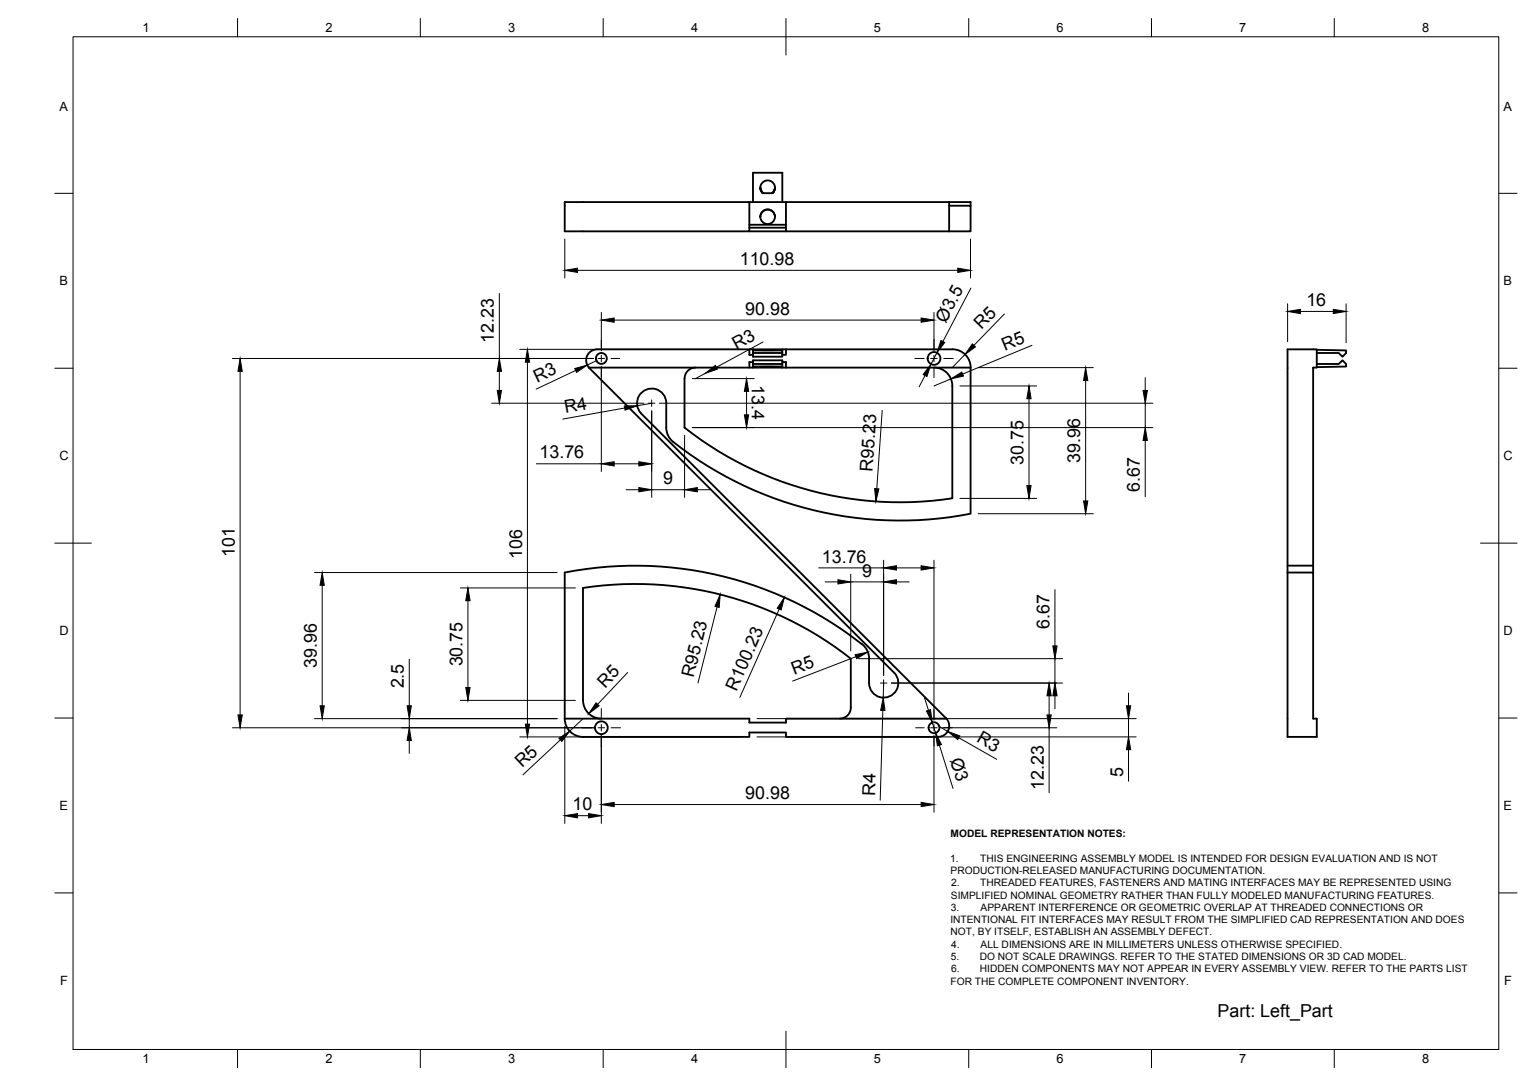
ISO-10303-21;
HEADER;
/* Generated by software containing ST-Developer
 * from STEP Tools, Inc. (www.steptools.com) 
 */

FILE_DESCRIPTION(
/* description */ (''),
/* implementation_level */ '2;1');

FILE_NAME(
/* name */ 'Left_Part.step',
/* time_stamp */ '2026-10-05T13:12:53-07:00',
/* author */ (''),
/* organization */ (''),
/* preprocessor_version */ 'ST-DEVELOPER v20.2',
/* originating_system */ 'Autodesk Translation Framework v15.15.0.0',
/* authorisation */ '');

FILE_SCHEMA (('AUTOMOTIVE_DESIGN { 1 0 10303 214 3 1 1 }'));
ENDSEC;

DATA;
#10=MECHANICAL_DESIGN_GEOMETRIC_PRESENTATION_REPRESENTATION('',(#59),#5912);
#43=SHAPE_REPRESENTATION_RELATIONSHIP('SRR','None',#5944,#51);
#51=ADVANCED_BREP_SHAPE_REPRESENTATION('',(#67),#5904);
#59=STYLED_ITEM('',(#5993),#67);
#67=MANIFOLD_SOLID_BREP('Body1',#3470);
#75=FACE_BOUND('',#374,.T.);
#76=FACE_BOUND('',#375,.T.);
#77=FACE_BOUND('',#379,.T.);
#78=FACE_BOUND('',#419,.T.);
#79=FACE_BOUND('',#421,.T.);
#80=FACE_BOUND('',#427,.T.);
#81=FACE_BOUND('',#428,.T.);
#82=FACE_BOUND('',#432,.T.);
#83=FACE_BOUND('',#437,.T.);
#84=FACE_BOUND('',#441,.T.);
#85=FACE_BOUND('',#442,.T.);
#96=ELLIPSE('',#3572,2.00043399581457,2.);
#97=ELLIPSE('',#3573,2.00173692551084,2.);
#98=ELLIPSE('',#3574,2.00173692551084,2.);
#99=ELLIPSE('',#3577,2.00043399581457,2.);
#100=ELLIPSE('',#3579,2.00043399581457,2.);
#101=ELLIPSE('',#3580,2.77129645175522,2.);
#102=ELLIPSE('',#3581,2.00043399581457,2.);
#103=ELLIPSE('',#3582,2.00043399581457,2.);
#114=CYLINDRICAL_SURFACE('',#3571,2.);
#115=CYLINDRICAL_SURFACE('',#3575,2.);
#116=CYLINDRICAL_SURFACE('',#3578,2.);
#117=CYLINDRICAL_SURFACE('',#3584,1.50000013517123);
#118=CYLINDRICAL_SURFACE('',#3588,1.4999996247669);
#119=CYLINDRICAL_SURFACE('',#3597,1.74999969554324);
#120=CYLINDRICAL_SURFACE('',#3601,4.99999999999999);
#121=CYLINDRICAL_SURFACE('',#3604,5.);
#122=CYLINDRICAL_SURFACE('',#3614,100.231846914414);
#123=CYLINDRICAL_SURFACE('',#3621,3.00000000000007);
#124=CYLINDRICAL_SURFACE('',#3625,95.2318469144141);
#125=CYLINDRICAL_SURFACE('',#3629,5.00000220964233);
#126=CYLINDRICAL_SURFACE('',#3633,3.99998589024062);
#127=CYLINDRICAL_SURFACE('',#3637,2.99999999999999);
#128=CYLINDRICAL_SURFACE('',#3640,3.00000000000001);
#129=CYLINDRICAL_SURFACE('',#3645,3.99998589024062);
#130=CYLINDRICAL_SURFACE('',#3649,5.00000220964233);
#131=CYLINDRICAL_SURFACE('',#3653,3.00000000000008);
#132=CYLINDRICAL_SURFACE('',#3656,2.99999999999999);
#133=CYLINDRICAL_SURFACE('',#3663,100.231846914414);
#134=CYLINDRICAL_SURFACE('',#3667,5.);
#135=CYLINDRICAL_SURFACE('',#3671,5.);
#136=CYLINDRICAL_SURFACE('',#3677,1.75000228959638);
#137=CYLINDRICAL_SURFACE('',#3694,95.231846914414);
#168=FACE_OUTER_BOUND('',#350,.T.);
#169=FACE_OUTER_BOUND('',#351,.T.);
#170=FACE_OUTER_BOUND('',#352,.T.);
#171=FACE_OUTER_BOUND('',#353,.T.);
#172=FACE_OUTER_BOUND('',#354,.T.);
#173=FACE_OUTER_BOUND('',#355,.T.);
#174=FACE_OUTER_BOUND('',#356,.T.);
#175=FACE_OUTER_BOUND('',#357,.T.);
#176=FACE_OUTER_BOUND('',#358,.T.);
#177=FACE_OUTER_BOUND('',#359,.T.);
#178=FACE_OUTER_BOUND('',#360,.T.);
#179=FACE_OUTER_BOUND('',#361,.T.);
#180=FACE_OUTER_BOUND('',#362,.T.);
#181=FACE_OUTER_BOUND('',#363,.T.);
#182=FACE_OUTER_BOUND('',#364,.T.);
#183=FACE_OUTER_BOUND('',#365,.T.);
#184=FACE_OUTER_BOUND('',#366,.T.);
#185=FACE_OUTER_BOUND('',#367,.T.);
#186=FACE_OUTER_BOUND('',#368,.T.);
#187=FACE_OUTER_BOUND('',#369,.T.);
#188=FACE_OUTER_BOUND('',#370,.T.);
#189=FACE_OUTER_BOUND('',#371,.T.);
#190=FACE_OUTER_BOUND('',#372,.T.);
#191=FACE_OUTER_BOUND('',#373,.T.);
#192=FACE_OUTER_BOUND('',#376,.T.);
#193=FACE_OUTER_BOUND('',#377,.T.);
#194=FACE_OUTER_BOUND('',#378,.T.);
#195=FACE_OUTER_BOUND('',#380,.T.);
#196=FACE_OUTER_BOUND('',#381,.T.);
#197=FACE_OUTER_BOUND('',#382,.T.);
#198=FACE_OUTER_BOUND('',#383,.T.);
#199=FACE_OUTER_BOUND('',#384,.T.);
#200=FACE_OUTER_BOUND('',#385,.T.);
#201=FACE_OUTER_BOUND('',#386,.T.);
#202=FACE_OUTER_BOUND('',#387,.T.);
#203=FACE_OUTER_BOUND('',#388,.T.);
#204=FACE_OUTER_BOUND('',#389,.T.);
#205=FACE_OUTER_BOUND('',#390,.T.);
#206=FACE_OUTER_BOUND('',#391,.T.);
#207=FACE_OUTER_BOUND('',#392,.T.);
#208=FACE_OUTER_BOUND('',#393,.T.);
#209=FACE_OUTER_BOUND('',#394,.T.);
#210=FACE_OUTER_BOUND('',#395,.T.);
#211=FACE_OUTER_BOUND('',#396,.T.);
#212=FACE_OUTER_BOUND('',#397,.T.);
#213=FACE_OUTER_BOUND('',#398,.T.);
#214=FACE_OUTER_BOUND('',#399,.T.);
#215=FACE_OUTER_BOUND('',#400,.T.);
#216=FACE_OUTER_BOUND('',#401,.T.);
#217=FACE_OUTER_BOUND('',#402,.T.);
#218=FACE_OUTER_BOUND('',#403,.T.);
#219=FACE_OUTER_BOUND('',#404,.T.);
#220=FACE_OUTER_BOUND('',#405,.T.);
#221=FACE_OUTER_BOUND('',#406,.T.);
#222=FACE_OUTER_BOUND('',#407,.T.);
#223=FACE_OUTER_BOUND('',#408,.T.);
#224=FACE_OUTER_BOUND('',#409,.T.);
#225=FACE_OUTER_BOUND('',#410,.T.);
#226=FACE_OUTER_BOUND('',#411,.T.);
#227=FACE_OUTER_BOUND('',#412,.T.);
#228=FACE_OUTER_BOUND('',#413,.T.);
#229=FACE_OUTER_BOUND('',#414,.T.);
#230=FACE_OUTER_BOUND('',#415,.T.);
#231=FACE_OUTER_BOUND('',#416,.T.);
#232=FACE_OUTER_BOUND('',#417,.T.);
#233=FACE_OUTER_BOUND('',#418,.T.);
#234=FACE_OUTER_BOUND('',#420,.T.);
#235=FACE_OUTER_BOUND('',#422,.T.);
#236=FACE_OUTER_BOUND('',#423,.T.);
#237=FACE_OUTER_BOUND('',#424,.T.);
#238=FACE_OUTER_BOUND('',#425,.T.);
#239=FACE_OUTER_BOUND('',#426,.T.);
#240=FACE_OUTER_BOUND('',#429,.T.);
#241=FACE_OUTER_BOUND('',#430,.T.);
#242=FACE_OUTER_BOUND('',#431,.T.);
#243=FACE_OUTER_BOUND('',#433,.T.);
#244=FACE_OUTER_BOUND('',#434,.T.);
#245=FACE_OUTER_BOUND('',#435,.T.);
#246=FACE_OUTER_BOUND('',#436,.T.);
#247=FACE_OUTER_BOUND('',#438,.T.);
#248=FACE_OUTER_BOUND('',#439,.T.);
#249=FACE_OUTER_BOUND('',#440,.T.);
#350=EDGE_LOOP('',(#2190,#2191));
#351=EDGE_LOOP('',(#2192,#2193,#2194,#2195,#2196,#2197));
#352=EDGE_LOOP('',(#2198,#2199,#2200,#2201));
#353=EDGE_LOOP('',(#2202,#2203,#2204,#2205,#2206,#2207));
#354=EDGE_LOOP('',(#2208,#2209,#2210,#2211,#2212,#2213,#2214));
#355=EDGE_LOOP('',(#2215,#2216,#2217,#2218));
#356=EDGE_LOOP('',(#2219));
#357=EDGE_LOOP('',(#2220,#2221,#2222,#2223));
#358=EDGE_LOOP('',(#2224));
#359=EDGE_LOOP('',(#2225,#2226,#2227,#2228,#2229,#2230));
#360=EDGE_LOOP('',(#2231,#2232,#2233,#2234,#2235,#2236));
#361=EDGE_LOOP('',(#2237,#2238,#2239,#2240,#2241));
#362=EDGE_LOOP('',(#2242));
#363=EDGE_LOOP('',(#2243,#2244,#2245,#2246));
#364=EDGE_LOOP('',(#2247,#2248,#2249,#2250,#2251,#2252));
#365=EDGE_LOOP('',(#2253,#2254,#2255,#2256));
#366=EDGE_LOOP('',(#2257,#2258,#2259,#2260));
#367=EDGE_LOOP('',(#2261,#2262,#2263,#2264,#2265,#2266));
#368=EDGE_LOOP('',(#2267,#2268,#2269,#2270));
#369=EDGE_LOOP('',(#2271,#2272,#2273,#2274));
#370=EDGE_LOOP('',(#2275,#2276,#2277,#2278));
#371=EDGE_LOOP('',(#2279,#2280,#2281,#2282,#2283,#2284));
#372=EDGE_LOOP('',(#2285,#2286,#2287,#2288));
#373=EDGE_LOOP('',(#2289,#2290,#2291,#2292,#2293,#2294,#2295,#2296,#2297,
#2298,#2299,#2300));
#374=EDGE_LOOP('',(#2301));
#375=EDGE_LOOP('',(#2302));
#376=EDGE_LOOP('',(#2303,#2304,#2305,#2306));
#377=EDGE_LOOP('',(#2307,#2308,#2309,#2310,#2311,#2312));
#378=EDGE_LOOP('',(#2313,#2314,#2315,#2316));
#379=EDGE_LOOP('',(#2317));
#380=EDGE_LOOP('',(#2318,#2319,#2320,#2321,#2322,#2323));
#381=EDGE_LOOP('',(#2324,#2325,#2326,#2327,#2328,#2329));
#382=EDGE_LOOP('',(#2330,#2331,#2332,#2333));
#383=EDGE_LOOP('',(#2334,#2335,#2336,#2337));
#384=EDGE_LOOP('',(#2338,#2339,#2340,#2341));
#385=EDGE_LOOP('',(#2342,#2343,#2344,#2345));
#386=EDGE_LOOP('',(#2346,#2347,#2348,#2349));
#387=EDGE_LOOP('',(#2350,#2351,#2352,#2353));
#388=EDGE_LOOP('',(#2354,#2355,#2356,#2357));
#389=EDGE_LOOP('',(#2358,#2359,#2360,#2361,#2362));
#390=EDGE_LOOP('',(#2363,#2364,#2365,#2366,#2367,#2368,#2369));
#391=EDGE_LOOP('',(#2370,#2371,#2372,#2373,#2374));
#392=EDGE_LOOP('',(#2375,#2376,#2377,#2378));
#393=EDGE_LOOP('',(#2379,#2380,#2381,#2382));
#394=EDGE_LOOP('',(#2383,#2384,#2385,#2386));
#395=EDGE_LOOP('',(#2387,#2388,#2389,#2390));
#396=EDGE_LOOP('',(#2391,#2392,#2393,#2394));
#397=EDGE_LOOP('',(#2395,#2396,#2397,#2398));
#398=EDGE_LOOP('',(#2399,#2400,#2401,#2402));
#399=EDGE_LOOP('',(#2403,#2404,#2405,#2406));
#400=EDGE_LOOP('',(#2407,#2408,#2409,#2410));
#401=EDGE_LOOP('',(#2411,#2412,#2413,#2414,#2415,#2416));
#402=EDGE_LOOP('',(#2417,#2418,#2419,#2420,#2421,#2422));
#403=EDGE_LOOP('',(#2423,#2424,#2425,#2426));
#404=EDGE_LOOP('',(#2427,#2428,#2429,#2430));
#405=EDGE_LOOP('',(#2431,#2432,#2433,#2434));
#406=EDGE_LOOP('',(#2435,#2436,#2437,#2438,#2439));
#407=EDGE_LOOP('',(#2440,#2441,#2442,#2443,#2444,#2445,#2446,#2447,#2448,
#2449,#2450));
#408=EDGE_LOOP('',(#2451,#2452,#2453,#2454));
#409=EDGE_LOOP('',(#2455,#2456,#2457,#2458));
#410=EDGE_LOOP('',(#2459,#2460,#2461,#2462,#2463,#2464,#2465,#2466,#2467,
#2468,#2469,#2470,#2471,#2472,#2473,#2474,#2475,#2476,#2477,#2478,#2479,
#2480,#2481,#2482,#2483,#2484,#2485,#2486,#2487));
#411=EDGE_LOOP('',(#2488,#2489,#2490,#2491));
#412=EDGE_LOOP('',(#2492));
#413=EDGE_LOOP('',(#2493,#2494,#2495,#2496));
#414=EDGE_LOOP('',(#2497,#2498,#2499,#2500,#2501,#2502,#2503,#2504));
#415=EDGE_LOOP('',(#2505,#2506,#2507,#2508));
#416=EDGE_LOOP('',(#2509,#2510,#2511,#2512));
#417=EDGE_LOOP('',(#2513,#2514,#2515,#2516));
#418=EDGE_LOOP('',(#2517,#2518,#2519,#2520));
#419=EDGE_LOOP('',(#2521));
#420=EDGE_LOOP('',(#2522,#2523,#2524,#2525));
#421=EDGE_LOOP('',(#2526));
#422=EDGE_LOOP('',(#2527,#2528,#2529,#2530));
#423=EDGE_LOOP('',(#2531,#2532,#2533,#2534));
#424=EDGE_LOOP('',(#2535,#2536,#2537,#2538,#2539,#2540));
#425=EDGE_LOOP('',(#2541,#2542,#2543,#2544,#2545,#2546));
#426=EDGE_LOOP('',(#2547,#2548,#2549,#2550,#2551,#2552,#2553,#2554,#2555,
#2556,#2557,#2558,#2559,#2560,#2561,#2562,#2563,#2564,#2565,#2566,#2567,
#2568,#2569));
#427=EDGE_LOOP('',(#2570,#2571,#2572,#2573,#2574,#2575,#2576,#2577,#2578,
#2579));
#428=EDGE_LOOP('',(#2580,#2581,#2582,#2583,#2584,#2585));
#429=EDGE_LOOP('',(#2586,#2587,#2588,#2589));
#430=EDGE_LOOP('',(#2590,#2591,#2592,#2593,#2594,#2595,#2596,#2597,#2598,
#2599,#2600,#2601,#2602,#2603));
#431=EDGE_LOOP('',(#2604,#2605,#2606,#2607));
#432=EDGE_LOOP('',(#2608,#2609,#2610));
#433=EDGE_LOOP('',(#2611,#2612,#2613,#2614));
#434=EDGE_LOOP('',(#2615,#2616,#2617,#2618));
#435=EDGE_LOOP('',(#2619,#2620,#2621,#2622));
#436=EDGE_LOOP('',(#2623,#2624,#2625,#2626));
#437=EDGE_LOOP('',(#2627));
#438=EDGE_LOOP('',(#2628,#2629,#2630,#2631,#2632,#2633,#2634,#2635));
#439=EDGE_LOOP('',(#2636,#2637,#2638,#2639));
#440=EDGE_LOOP('',(#2640,#2641,#2642,#2643,#2644,#2645,#2646,#2647,#2648,
#2649,#2650,#2651));
#441=EDGE_LOOP('',(#2652));
#442=EDGE_LOOP('',(#2653));
#553=CIRCLE('',#3570,2.);
#554=CIRCLE('',#3576,2.);
#555=CIRCLE('',#3585,1.50000013517123);
#556=CIRCLE('',#3586,1.50000013517123);
#557=CIRCLE('',#3589,1.4999996247669);
#558=CIRCLE('',#3590,1.4999996247669);
#559=CIRCLE('',#3596,1.74999969554324);
#560=CIRCLE('',#3598,1.74999969554324);
#561=CIRCLE('',#3602,4.99999999999999);
#562=CIRCLE('',#3603,4.99999999999999);
#563=CIRCLE('',#3605,5.);
#564=CIRCLE('',#3606,5.);
#565=CIRCLE('',#3613,2.99999999999999);
#566=CIRCLE('',#3615,100.231846914414);
#567=CIRCLE('',#3616,100.231846914414);
#568=CIRCLE('',#3622,3.00000000000007);
#569=CIRCLE('',#3623,3.00000000000007);
#570=CIRCLE('',#3626,95.2318469144141);
#571=CIRCLE('',#3627,95.2318469144141);
#572=CIRCLE('',#3630,5.00000220964233);
#573=CIRCLE('',#3631,5.00000220964233);
#574=CIRCLE('',#3634,3.99998589024062);
#575=CIRCLE('',#3635,3.99998589024062);
#576=CIRCLE('',#3638,2.99999999999999);
#577=CIRCLE('',#3639,2.99999999999999);
#578=CIRCLE('',#3641,3.00000000000001);
#579=CIRCLE('',#3642,3.00000000000001);
#580=CIRCLE('',#3643,3.00000000000001);
#581=CIRCLE('',#3646,3.99998589024062);
#582=CIRCLE('',#3647,3.99998589024062);
#583=CIRCLE('',#3650,5.00000220964233);
#584=CIRCLE('',#3651,5.00000220964233);
#585=CIRCLE('',#3654,3.00000000000008);
#586=CIRCLE('',#3655,3.00000000000008);
#587=CIRCLE('',#3657,2.99999999999999);
#588=CIRCLE('',#3664,100.231846914414);
#589=CIRCLE('',#3665,100.231846914414);
#590=CIRCLE('',#3668,5.);
#591=CIRCLE('',#3669,5.);
#592=CIRCLE('',#3672,5.);
#593=CIRCLE('',#3673,5.);
#594=CIRCLE('',#3676,95.231846914414);
#595=CIRCLE('',#3678,1.75000228959638);
#596=CIRCLE('',#3679,1.75000228959638);
#597=CIRCLE('',#3693,95.231846914414);
#655=LINE('',#4894,#1020);
#656=LINE('',#4900,#1021);
#657=LINE('',#4907,#1022);
#658=LINE('',#4917,#1023);
#659=LINE('',#4921,#1024);
#660=LINE('',#4923,#1025);
#661=LINE('',#4925,#1026);
#662=LINE('',#4927,#1027);
#663=LINE('',#4928,#1028);
#664=LINE('',#4933,#1029);
#665=LINE('',#4940,#1030);
#666=LINE('',#4945,#1031);
#667=LINE('',#4947,#1032);
#668=LINE('',#4949,#1033);
#669=LINE('',#4951,#1034);
#670=LINE('',#4952,#1035);
#671=LINE('',#4956,#1036);
#672=LINE('',#4958,#1037);
#673=LINE('',#4960,#1038);
#674=LINE('',#4962,#1039);
#675=LINE('',#4964,#1040);
#676=LINE('',#4965,#1041);
#677=LINE('',#4968,#1042);
#678=LINE('',#4970,#1043);
#679=LINE('',#4972,#1044);
#680=LINE('',#4973,#1045);
#681=LINE('',#4979,#1046);
#682=LINE('',#4983,#1047);
#683=LINE('',#4985,#1048);
#684=LINE('',#4987,#1049);
#685=LINE('',#4989,#1050);
#686=LINE('',#4990,#1051);
#687=LINE('',#4994,#1052);
#688=LINE('',#4996,#1053);
#689=LINE('',#4998,#1054);
#690=LINE('',#4999,#1055);
#691=LINE('',#5007,#1056);
#692=LINE('',#5010,#1057);
#693=LINE('',#5012,#1058);
#694=LINE('',#5013,#1059);
#695=LINE('',#5016,#1060);
#696=LINE('',#5018,#1061);
#697=LINE('',#5019,#1062);
#698=LINE('',#5022,#1063);
#699=LINE('',#5023,#1064);
#700=LINE('',#5026,#1065);
#701=LINE('',#5027,#1066);
#702=LINE('',#5030,#1067);
#703=LINE('',#5031,#1068);
#704=LINE('',#5034,#1069);
#705=LINE('',#5036,#1070);
#706=LINE('',#5038,#1071);
#707=LINE('',#5042,#1072);
#708=LINE('',#5043,#1073);
#709=LINE('',#5048,#1074);
#710=LINE('',#5052,#1075);
#711=LINE('',#5053,#1076);
#712=LINE('',#5055,#1077);
#713=LINE('',#5058,#1078);
#714=LINE('',#5059,#1079);
#715=LINE('',#5062,#1080);
#716=LINE('',#5064,#1081);
#717=LINE('',#5066,#1082);
#718=LINE('',#5067,#1083);
#719=LINE('',#5073,#1084);
#720=LINE('',#5076,#1085);
#721=LINE('',#5078,#1086);
#722=LINE('',#5079,#1087);
#723=LINE('',#5085,#1088);
#724=LINE('',#5087,#1089);
#725=LINE('',#5088,#1090);
#726=LINE('',#5094,#1091);
#727=LINE('',#5097,#1092);
#728=LINE('',#5099,#1093);
#729=LINE('',#5100,#1094);
#730=LINE('',#5106,#1095);
#731=LINE('',#5109,#1096);
#732=LINE('',#5111,#1097);
#733=LINE('',#5112,#1098);
#734=LINE('',#5117,#1099);
#735=LINE('',#5124,#1100);
#736=LINE('',#5129,#1101);
#737=LINE('',#5132,#1102);
#738=LINE('',#5134,#1103);
#739=LINE('',#5135,#1104);
#740=LINE('',#5140,#1105);
#741=LINE('',#5144,#1106);
#742=LINE('',#5146,#1107);
#743=LINE('',#5147,#1108);
#744=LINE('',#5152,#1109);
#745=LINE('',#5157,#1110);
#746=LINE('',#5159,#1111);
#747=LINE('',#5161,#1112);
#748=LINE('',#5162,#1113);
#749=LINE('',#5167,#1114);
#750=LINE('',#5171,#1115);
#751=LINE('',#5174,#1116);
#752=LINE('',#5178,#1117);
#753=LINE('',#5180,#1118);
#754=LINE('',#5182,#1119);
#755=LINE('',#5183,#1120);
#756=LINE('',#5187,#1121);
#757=LINE('',#5189,#1122);
#758=LINE('',#5191,#1123);
#759=LINE('',#5192,#1124);
#760=LINE('',#5196,#1125);
#761=LINE('',#5198,#1126);
#762=LINE('',#5200,#1127);
#763=LINE('',#5202,#1128);
#764=LINE('',#5204,#1129);
#765=LINE('',#5205,#1130);
#766=LINE('',#5209,#1131);
#767=LINE('',#5211,#1132);
#768=LINE('',#5213,#1133);
#769=LINE('',#5215,#1134);
#770=LINE('',#5217,#1135);
#771=LINE('',#5218,#1136);
#772=LINE('',#5220,#1137);
#773=LINE('',#5221,#1138);
#774=LINE('',#5226,#1139);
#775=LINE('',#5230,#1140);
#776=LINE('',#5232,#1141);
#777=LINE('',#5233,#1142);
#778=LINE('',#5238,#1143);
#779=LINE('',#5241,#1144);
#780=LINE('',#5244,#1145);
#781=LINE('',#5246,#1146);
#782=LINE('',#5248,#1147);
#783=LINE('',#5249,#1148);
#784=LINE('',#5250,#1149);
#785=LINE('',#5251,#1150);
#786=LINE('',#5252,#1151);
#787=LINE('',#5258,#1152);
#788=LINE('',#5261,#1153);
#789=LINE('',#5264,#1154);
#790=LINE('',#5266,#1155);
#791=LINE('',#5267,#1156);
#792=LINE('',#5269,#1157);
#793=LINE('',#5271,#1158);
#794=LINE('',#5276,#1159);
#795=LINE('',#5282,#1160);
#796=LINE('',#5284,#1161);
#797=LINE('',#5286,#1162);
#798=LINE('',#5287,#1163);
#799=LINE('',#5290,#1164);
#800=LINE('',#5291,#1165);
#801=LINE('',#5293,#1166);
#802=LINE('',#5294,#1167);
#803=LINE('',#5297,#1168);
#804=LINE('',#5298,#1169);
#805=LINE('',#5300,#1170);
#806=LINE('',#5303,#1171);
#807=LINE('',#5305,#1172);
#808=LINE('',#5306,#1173);
#809=LINE('',#5308,#1174);
#810=LINE('',#5311,#1175);
#811=LINE('',#5312,#1176);
#812=LINE('',#5315,#1177);
#813=LINE('',#5316,#1178);
#814=LINE('',#5318,#1179);
#815=LINE('',#5323,#1180);
#816=LINE('',#5325,#1181);
#817=LINE('',#5327,#1182);
#818=LINE('',#5329,#1183);
#819=LINE('',#5331,#1184);
#820=LINE('',#5332,#1185);
#821=LINE('',#5335,#1186);
#822=LINE('',#5338,#1187);
#823=LINE('',#5339,#1188);
#824=LINE('',#5340,#1189);
#825=LINE('',#5341,#1190);
#826=LINE('',#5342,#1191);
#827=LINE('',#5344,#1192);
#828=LINE('',#5346,#1193);
#829=LINE('',#5348,#1194);
#830=LINE('',#5350,#1195);
#831=LINE('',#5352,#1196);
#832=LINE('',#5354,#1197);
#833=LINE('',#5356,#1198);
#1020=VECTOR('',#3892,10.);
#1021=VECTOR('',#3899,2.);
#1022=VECTOR('',#3908,2.);
#1023=VECTOR('',#3919,2.);
#1024=VECTOR('',#3924,10.);
#1025=VECTOR('',#3925,10.);
#1026=VECTOR('',#3926,10.);
#1027=VECTOR('',#3927,10.);
#1028=VECTOR('',#3928,10.);
#1029=VECTOR('',#3933,1.50000013517123);
#1030=VECTOR('',#3942,1.4999996247669);
#1031=VECTOR('',#3949,10.);
#1032=VECTOR('',#3950,10.);
#1033=VECTOR('',#3951,10.);
#1034=VECTOR('',#3952,10.);
#1035=VECTOR('',#3953,10.);
#1036=VECTOR('',#3956,10.);
#1037=VECTOR('',#3957,10.);
#1038=VECTOR('',#3958,10.);
#1039=VECTOR('',#3959,10.);
#1040=VECTOR('',#3960,10.);
#1041=VECTOR('',#3961,10.);
#1042=VECTOR('',#3964,10.);
#1043=VECTOR('',#3965,10.);
#1044=VECTOR('',#3966,10.);
#1045=VECTOR('',#3967,10.);
#1046=VECTOR('',#3974,1.74999969554324);
#1047=VECTOR('',#3979,10.);
#1048=VECTOR('',#3980,10.);
#1049=VECTOR('',#3981,10.);
#1050=VECTOR('',#3982,10.);
#1051=VECTOR('',#3983,10.);
#1052=VECTOR('',#3986,10.);
#1053=VECTOR('',#3987,10.);
#1054=VECTOR('',#3988,10.);
#1055=VECTOR('',#3989,10.);
#1056=VECTOR('',#4002,10.);
#1057=VECTOR('',#4005,10.);
#1058=VECTOR('',#4006,10.);
#1059=VECTOR('',#4007,10.);
#1060=VECTOR('',#4010,10.);
#1061=VECTOR('',#4011,10.);
#1062=VECTOR('',#4012,10.);
#1063=VECTOR('',#4015,10.);
#1064=VECTOR('',#4016,10.);
#1065=VECTOR('',#4019,10.);
#1066=VECTOR('',#4020,10.);
#1067=VECTOR('',#4023,10.);
#1068=VECTOR('',#4024,10.);
#1069=VECTOR('',#4027,10.);
#1070=VECTOR('',#4028,10.);
#1071=VECTOR('',#4029,10.);
#1072=VECTOR('',#4032,10.);
#1073=VECTOR('',#4033,10.);
#1074=VECTOR('',#4038,10.);
#1075=VECTOR('',#4043,10.);
#1076=VECTOR('',#4044,10.);
#1077=VECTOR('',#4047,10.);
#1078=VECTOR('',#4050,10.);
#1079=VECTOR('',#4051,10.);
#1080=VECTOR('',#4054,10.);
#1081=VECTOR('',#4055,10.);
#1082=VECTOR('',#4056,10.);
#1083=VECTOR('',#4057,10.);
#1084=VECTOR('',#4064,10.);
#1085=VECTOR('',#4067,9.99999999999999);
#1086=VECTOR('',#4068,9.99999999999999);
#1087=VECTOR('',#4069,10.);
#1088=VECTOR('',#4078,10.);
#1089=VECTOR('',#4079,10.);
#1090=VECTOR('',#4080,10.);
#1091=VECTOR('',#4087,10.);
#1092=VECTOR('',#4090,10.);
#1093=VECTOR('',#4091,10.);
#1094=VECTOR('',#4092,10.);
#1095=VECTOR('',#4099,10.);
#1096=VECTOR('',#4102,10.);
#1097=VECTOR('',#4103,10.);
#1098=VECTOR('',#4104,10.);
#1099=VECTOR('',#4109,10.);
#1100=VECTOR('',#4116,10.);
#1101=VECTOR('',#4121,10.);
#1102=VECTOR('',#4124,10.);
#1103=VECTOR('',#4125,10.);
#1104=VECTOR('',#4126,10.);
#1105=VECTOR('',#4131,10.);
#1106=VECTOR('',#4136,10.);
#1107=VECTOR('',#4137,10.);
#1108=VECTOR('',#4138,10.);
#1109=VECTOR('',#4143,10.);
#1110=VECTOR('',#4148,9.99999999999999);
#1111=VECTOR('',#4149,10.);
#1112=VECTOR('',#4150,9.99999999999999);
#1113=VECTOR('',#4151,10.);
#1114=VECTOR('',#4156,10.);
#1115=VECTOR('',#4161,10.);
#1116=VECTOR('',#4164,10.);
#1117=VECTOR('',#4167,10.);
#1118=VECTOR('',#4168,10.);
#1119=VECTOR('',#4169,10.);
#1120=VECTOR('',#4170,10.);
#1121=VECTOR('',#4173,10.);
#1122=VECTOR('',#4174,10.);
#1123=VECTOR('',#4175,10.);
#1124=VECTOR('',#4176,10.);
#1125=VECTOR('',#4179,10.);
#1126=VECTOR('',#4180,10.);
#1127=VECTOR('',#4181,10.);
#1128=VECTOR('',#4182,10.);
#1129=VECTOR('',#4183,10.);
#1130=VECTOR('',#4184,10.);
#1131=VECTOR('',#4187,10.);
#1132=VECTOR('',#4188,10.);
#1133=VECTOR('',#4189,10.);
#1134=VECTOR('',#4190,10.);
#1135=VECTOR('',#4191,10.);
#1136=VECTOR('',#4192,10.);
#1137=VECTOR('',#4195,10.);
#1138=VECTOR('',#4196,10.);
#1139=VECTOR('',#4201,10.);
#1140=VECTOR('',#4206,10.);
#1141=VECTOR('',#4207,10.);
#1142=VECTOR('',#4208,10.);
#1143=VECTOR('',#4213,10.);
#1144=VECTOR('',#4216,10.);
#1145=VECTOR('',#4219,10.);
#1146=VECTOR('',#4220,10.);
#1147=VECTOR('',#4221,10.);
#1148=VECTOR('',#4222,10.);
#1149=VECTOR('',#4223,10.);
#1150=VECTOR('',#4224,10.);
#1151=VECTOR('',#4225,10.);
#1152=VECTOR('',#4230,10.);
#1153=VECTOR('',#4233,10.);
#1154=VECTOR('',#4236,10.);
#1155=VECTOR('',#4237,10.);
#1156=VECTOR('',#4238,10.);
#1157=VECTOR('',#4241,10.);
#1158=VECTOR('',#4244,10.);
#1159=VECTOR('',#4249,1.75000228959638);
#1160=VECTOR('',#4256,10.);
#1161=VECTOR('',#4257,10.);
#1162=VECTOR('',#4258,10.);
#1163=VECTOR('',#4259,10.);
#1164=VECTOR('',#4262,10.);
#1165=VECTOR('',#4263,10.);
#1166=VECTOR('',#4264,10.);
#1167=VECTOR('',#4265,10.);
#1168=VECTOR('',#4268,10.);
#1169=VECTOR('',#4269,10.);
#1170=VECTOR('',#4272,10.);
#1171=VECTOR('',#4275,10.);
#1172=VECTOR('',#4276,10.);
#1173=VECTOR('',#4277,10.);
#1174=VECTOR('',#4280,10.);
#1175=VECTOR('',#4283,10.);
#1176=VECTOR('',#4284,10.);
#1177=VECTOR('',#4287,10.);
#1178=VECTOR('',#4288,10.);
#1179=VECTOR('',#4291,10.);
#1180=VECTOR('',#4296,10.);
#1181=VECTOR('',#4297,10.);
#1182=VECTOR('',#4298,10.);
#1183=VECTOR('',#4299,10.);
#1184=VECTOR('',#4300,10.);
#1185=VECTOR('',#4301,10.);
#1186=VECTOR('',#4306,10.);
#1187=VECTOR('',#4311,10.);
#1188=VECTOR('',#4312,10.);
#1189=VECTOR('',#4313,10.);
#1190=VECTOR('',#4314,10.);
#1191=VECTOR('',#4315,10.);
#1192=VECTOR('',#4318,10.);
#1193=VECTOR('',#4321,10.);
#1194=VECTOR('',#4324,10.);
#1195=VECTOR('',#4327,10.);
#1196=VECTOR('',#4330,10.);
#1197=VECTOR('',#4333,10.);
#1198=VECTOR('',#4336,10.);
#1385=VERTEX_POINT('',#4892);
#1386=VERTEX_POINT('',#4893);
#1387=VERTEX_POINT('',#4897);
#1388=VERTEX_POINT('',#4899);
#1389=VERTEX_POINT('',#4904);
#1390=VERTEX_POINT('',#4906);
#1391=VERTEX_POINT('',#4910);
#1392=VERTEX_POINT('',#4911);
#1393=VERTEX_POINT('',#4913);
#1394=VERTEX_POINT('',#4916);
#1395=VERTEX_POINT('',#4920);
#1396=VERTEX_POINT('',#4922);
#1397=VERTEX_POINT('',#4924);
#1398=VERTEX_POINT('',#4926);
#1399=VERTEX_POINT('',#4930);
#1400=VERTEX_POINT('',#4932);
#1401=VERTEX_POINT('',#4937);
#1402=VERTEX_POINT('',#4939);
#1403=VERTEX_POINT('',#4944);
#1404=VERTEX_POINT('',#4946);
#1405=VERTEX_POINT('',#4948);
#1406=VERTEX_POINT('',#4950);
#1407=VERTEX_POINT('',#4954);
#1408=VERTEX_POINT('',#4955);
#1409=VERTEX_POINT('',#4957);
#1410=VERTEX_POINT('',#4959);
#1411=VERTEX_POINT('',#4961);
#1412=VERTEX_POINT('',#4963);
#1413=VERTEX_POINT('',#4967);
#1414=VERTEX_POINT('',#4969);
#1415=VERTEX_POINT('',#4971);
#1416=VERTEX_POINT('',#4975);
#1417=VERTEX_POINT('',#4978);
#1418=VERTEX_POINT('',#4982);
#1419=VERTEX_POINT('',#4984);
#1420=VERTEX_POINT('',#4986);
#1421=VERTEX_POINT('',#4988);
#1422=VERTEX_POINT('',#4992);
#1423=VERTEX_POINT('',#4993);
#1424=VERTEX_POINT('',#4995);
#1425=VERTEX_POINT('',#4997);
#1426=VERTEX_POINT('',#5004);
#1427=VERTEX_POINT('',#5009);
#1428=VERTEX_POINT('',#5011);
#1429=VERTEX_POINT('',#5015);
#1430=VERTEX_POINT('',#5017);
#1431=VERTEX_POINT('',#5021);
#1432=VERTEX_POINT('',#5025);
#1433=VERTEX_POINT('',#5029);
#1434=VERTEX_POINT('',#5033);
#1435=VERTEX_POINT('',#5035);
#1436=VERTEX_POINT('',#5037);
#1437=VERTEX_POINT('',#5039);
#1438=VERTEX_POINT('',#5041);
#1439=VERTEX_POINT('',#5045);
#1440=VERTEX_POINT('',#5047);
#1441=VERTEX_POINT('',#5051);
#1442=VERTEX_POINT('',#5057);
#1443=VERTEX_POINT('',#5061);
#1444=VERTEX_POINT('',#5063);
#1445=VERTEX_POINT('',#5065);
#1446=VERTEX_POINT('',#5069);
#1447=VERTEX_POINT('',#5071);
#1448=VERTEX_POINT('',#5075);
#1449=VERTEX_POINT('',#5077);
#1450=VERTEX_POINT('',#5084);
#1451=VERTEX_POINT('',#5086);
#1452=VERTEX_POINT('',#5090);
#1453=VERTEX_POINT('',#5092);
#1454=VERTEX_POINT('',#5096);
#1455=VERTEX_POINT('',#5098);
#1456=VERTEX_POINT('',#5102);
#1457=VERTEX_POINT('',#5104);
#1458=VERTEX_POINT('',#5108);
#1459=VERTEX_POINT('',#5110);
#1460=VERTEX_POINT('',#5114);
#1461=VERTEX_POINT('',#5116);
#1462=VERTEX_POINT('',#5120);
#1463=VERTEX_POINT('',#5121);
#1464=VERTEX_POINT('',#5123);
#1465=VERTEX_POINT('',#5125);
#1466=VERTEX_POINT('',#5127);
#1467=VERTEX_POINT('',#5131);
#1468=VERTEX_POINT('',#5133);
#1469=VERTEX_POINT('',#5137);
#1470=VERTEX_POINT('',#5139);
#1471=VERTEX_POINT('',#5143);
#1472=VERTEX_POINT('',#5145);
#1473=VERTEX_POINT('',#5149);
#1474=VERTEX_POINT('',#5151);
#1475=VERTEX_POINT('',#5155);
#1476=VERTEX_POINT('',#5156);
#1477=VERTEX_POINT('',#5158);
#1478=VERTEX_POINT('',#5160);
#1479=VERTEX_POINT('',#5164);
#1480=VERTEX_POINT('',#5166);
#1481=VERTEX_POINT('',#5170);
#1482=VERTEX_POINT('',#5172);
#1483=VERTEX_POINT('',#5176);
#1484=VERTEX_POINT('',#5177);
#1485=VERTEX_POINT('',#5179);
#1486=VERTEX_POINT('',#5181);
#1487=VERTEX_POINT('',#5185);
#1488=VERTEX_POINT('',#5186);
#1489=VERTEX_POINT('',#5188);
#1490=VERTEX_POINT('',#5190);
#1491=VERTEX_POINT('',#5194);
#1492=VERTEX_POINT('',#5195);
#1493=VERTEX_POINT('',#5197);
#1494=VERTEX_POINT('',#5199);
#1495=VERTEX_POINT('',#5201);
#1496=VERTEX_POINT('',#5203);
#1497=VERTEX_POINT('',#5207);
#1498=VERTEX_POINT('',#5208);
#1499=VERTEX_POINT('',#5210);
#1500=VERTEX_POINT('',#5212);
#1501=VERTEX_POINT('',#5214);
#1502=VERTEX_POINT('',#5216);
#1503=VERTEX_POINT('',#5223);
#1504=VERTEX_POINT('',#5225);
#1505=VERTEX_POINT('',#5229);
#1506=VERTEX_POINT('',#5231);
#1507=VERTEX_POINT('',#5235);
#1508=VERTEX_POINT('',#5237);
#1509=VERTEX_POINT('',#5239);
#1510=VERTEX_POINT('',#5243);
#1511=VERTEX_POINT('',#5245);
#1512=VERTEX_POINT('',#5247);
#1513=VERTEX_POINT('',#5254);
#1514=VERTEX_POINT('',#5255);
#1515=VERTEX_POINT('',#5257);
#1516=VERTEX_POINT('',#5259);
#1517=VERTEX_POINT('',#5263);
#1518=VERTEX_POINT('',#5265);
#1519=VERTEX_POINT('',#5273);
#1520=VERTEX_POINT('',#5275);
#1521=VERTEX_POINT('',#5280);
#1522=VERTEX_POINT('',#5281);
#1523=VERTEX_POINT('',#5283);
#1524=VERTEX_POINT('',#5285);
#1525=VERTEX_POINT('',#5289);
#1526=VERTEX_POINT('',#5292);
#1527=VERTEX_POINT('',#5296);
#1528=VERTEX_POINT('',#5302);
#1529=VERTEX_POINT('',#5304);
#1530=VERTEX_POINT('',#5310);
#1531=VERTEX_POINT('',#5314);
#1532=VERTEX_POINT('',#5321);
#1533=VERTEX_POINT('',#5322);
#1534=VERTEX_POINT('',#5324);
#1535=VERTEX_POINT('',#5326);
#1536=VERTEX_POINT('',#5328);
#1537=VERTEX_POINT('',#5330);
#1705=EDGE_CURVE('',#1385,#1386,#655,.T.);
#1706=EDGE_CURVE('',#1386,#1385,#553,.T.);
#1707=EDGE_CURVE('',#1387,#1387,#96,.T.);
#1708=EDGE_CURVE('',#1387,#1388,#656,.T.);
#1709=EDGE_CURVE('',#1386,#1388,#97,.T.);
#1710=EDGE_CURVE('',#1388,#1385,#98,.T.);
#1711=EDGE_CURVE('',#1389,#1389,#554,.T.);
#1712=EDGE_CURVE('',#1389,#1390,#657,.T.);
#1713=EDGE_CURVE('',#1390,#1390,#99,.T.);
#1714=EDGE_CURVE('',#1391,#1392,#100,.T.);
#1715=EDGE_CURVE('',#1393,#1391,#101,.T.);
#1716=EDGE_CURVE('',#1392,#1393,#102,.T.);
#1717=EDGE_CURVE('',#1392,#1394,#658,.T.);
#1718=EDGE_CURVE('',#1394,#1394,#103,.T.);
#1719=EDGE_CURVE('',#1393,#1395,#659,.T.);
#1720=EDGE_CURVE('',#1395,#1396,#660,.T.);
#1721=EDGE_CURVE('',#1397,#1396,#661,.T.);
#1722=EDGE_CURVE('',#1398,#1397,#662,.T.);
#1723=EDGE_CURVE('',#1398,#1391,#663,.T.);
#1724=EDGE_CURVE('',#1399,#1399,#555,.T.);
#1725=EDGE_CURVE('',#1399,#1400,#664,.T.);
#1726=EDGE_CURVE('',#1400,#1400,#556,.T.);
#1727=EDGE_CURVE('',#1401,#1401,#557,.T.);
#1728=EDGE_CURVE('',#1401,#1402,#665,.T.);
#1729=EDGE_CURVE('',#1402,#1402,#558,.T.);
#1730=EDGE_CURVE('',#1396,#1403,#666,.T.);
#1731=EDGE_CURVE('',#1404,#1395,#667,.T.);
#1732=EDGE_CURVE('',#1405,#1404,#668,.T.);
#1733=EDGE_CURVE('',#1406,#1405,#669,.T.);
#1734=EDGE_CURVE('',#1403,#1406,#670,.T.);
#1735=EDGE_CURVE('',#1407,#1408,#671,.T.);
#1736=EDGE_CURVE('',#1409,#1407,#672,.T.);
#1737=EDGE_CURVE('',#1410,#1409,#673,.T.);
#1738=EDGE_CURVE('',#1411,#1410,#674,.T.);
#1739=EDGE_CURVE('',#1412,#1411,#675,.T.);
#1740=EDGE_CURVE('',#1412,#1408,#676,.T.);
#1741=EDGE_CURVE('',#1413,#1407,#677,.T.);
#1742=EDGE_CURVE('',#1414,#1413,#678,.T.);
#1743=EDGE_CURVE('',#1415,#1414,#679,.T.);
#1744=EDGE_CURVE('',#1415,#1409,#680,.T.);
#1745=EDGE_CURVE('',#1416,#1416,#559,.T.);
#1746=EDGE_CURVE('',#1416,#1417,#681,.T.);
#1747=EDGE_CURVE('',#1417,#1417,#560,.T.);
#1748=EDGE_CURVE('',#1418,#1406,#682,.T.);
#1749=EDGE_CURVE('',#1418,#1419,#683,.T.);
#1750=EDGE_CURVE('',#1420,#1419,#684,.T.);
#1751=EDGE_CURVE('',#1420,#1421,#685,.T.);
#1752=EDGE_CURVE('',#1403,#1421,#686,.T.);
#1753=EDGE_CURVE('',#1422,#1423,#687,.T.);
#1754=EDGE_CURVE('',#1422,#1424,#688,.T.);
#1755=EDGE_CURVE('',#1425,#1424,#689,.T.);
#1756=EDGE_CURVE('',#1423,#1425,#690,.T.);
#1757=EDGE_CURVE('',#1423,#1418,#561,.T.);
#1758=EDGE_CURVE('',#1419,#1425,#562,.T.);
#1759=EDGE_CURVE('',#1415,#1426,#563,.T.);
#1760=EDGE_CURVE('',#1421,#1413,#564,.T.);
#1761=EDGE_CURVE('',#1426,#1420,#691,.T.);
#1762=EDGE_CURVE('',#1427,#1426,#692,.T.);
#1763=EDGE_CURVE('',#1428,#1420,#693,.T.);
#1764=EDGE_CURVE('',#1427,#1428,#694,.T.);
#1765=EDGE_CURVE('',#1429,#1410,#695,.T.);
#1766=EDGE_CURVE('',#1429,#1430,#696,.T.);
#1767=EDGE_CURVE('',#1430,#1411,#697,.T.);
#1768=EDGE_CURVE('',#1430,#1431,#698,.T.);
#1769=EDGE_CURVE('',#1412,#1431,#699,.T.);
#1770=EDGE_CURVE('',#1398,#1432,#700,.T.);
#1771=EDGE_CURVE('',#1432,#1404,#701,.T.);
#1772=EDGE_CURVE('',#1432,#1433,#702,.T.);
#1773=EDGE_CURVE('',#1405,#1433,#703,.T.);
#1774=EDGE_CURVE('',#1408,#1434,#704,.T.);
#1775=EDGE_CURVE('',#1434,#1435,#705,.T.);
#1776=EDGE_CURVE('',#1435,#1436,#706,.T.);
#1777=EDGE_CURVE('',#1436,#1437,#565,.T.);
#1778=EDGE_CURVE('',#1437,#1438,#707,.T.);
#1779=EDGE_CURVE('',#1438,#1397,#708,.T.);
#1780=EDGE_CURVE('',#1439,#1428,#566,.T.);
#1781=EDGE_CURVE('',#1440,#1439,#709,.T.);
#1782=EDGE_CURVE('',#1427,#1440,#567,.T.);
#1783=EDGE_CURVE('',#1441,#1438,#710,.T.);
#1784=EDGE_CURVE('',#1433,#1441,#711,.T.);
#1785=EDGE_CURVE('',#1431,#1434,#712,.T.);
#1786=EDGE_CURVE('',#1442,#1429,#713,.T.);
#1787=EDGE_CURVE('',#1435,#1442,#714,.T.);
#1788=EDGE_CURVE('',#1443,#1437,#715,.T.);
#1789=EDGE_CURVE('',#1444,#1443,#716,.T.);
#1790=EDGE_CURVE('',#1445,#1444,#717,.T.);
#1791=EDGE_CURVE('',#1441,#1445,#718,.T.);
#1792=EDGE_CURVE('',#1445,#1446,#568,.T.);
#1793=EDGE_CURVE('',#1447,#1444,#569,.T.);
#1794=EDGE_CURVE('',#1446,#1447,#719,.T.);
#1795=EDGE_CURVE('',#1446,#1448,#720,.T.);
#1796=EDGE_CURVE('',#1449,#1447,#721,.T.);
#1797=EDGE_CURVE('',#1448,#1449,#722,.T.);
#1798=EDGE_CURVE('',#1448,#1422,#570,.T.);
#1799=EDGE_CURVE('',#1424,#1449,#571,.T.);
#1800=EDGE_CURVE('',#1440,#1450,#723,.T.);
#1801=EDGE_CURVE('',#1451,#1439,#724,.T.);
#1802=EDGE_CURVE('',#1450,#1451,#725,.T.);
#1803=EDGE_CURVE('',#1450,#1452,#572,.T.);
#1804=EDGE_CURVE('',#1453,#1451,#573,.T.);
#1805=EDGE_CURVE('',#1452,#1453,#726,.T.);
#1806=EDGE_CURVE('',#1454,#1452,#727,.T.);
#1807=EDGE_CURVE('',#1455,#1453,#728,.T.);
#1808=EDGE_CURVE('',#1454,#1455,#729,.T.);
#1809=EDGE_CURVE('',#1456,#1454,#574,.T.);
#1810=EDGE_CURVE('',#1457,#1455,#575,.T.);
#1811=EDGE_CURVE('',#1457,#1456,#730,.T.);
#1812=EDGE_CURVE('',#1442,#1458,#731,.T.);
#1813=EDGE_CURVE('',#1458,#1459,#732,.T.);
#1814=EDGE_CURVE('',#1459,#1436,#733,.T.);
#1815=EDGE_CURVE('',#1460,#1458,#576,.T.);
#1816=EDGE_CURVE('',#1460,#1461,#734,.T.);
#1817=EDGE_CURVE('',#1443,#1461,#577,.T.);
#1818=EDGE_CURVE('',#1462,#1463,#578,.T.);
#1819=EDGE_CURVE('',#1462,#1464,#735,.T.);
#1820=EDGE_CURVE('',#1465,#1464,#579,.T.);
#1821=EDGE_CURVE('',#1466,#1465,#580,.T.);
#1822=EDGE_CURVE('',#1463,#1466,#736,.T.);
#1823=EDGE_CURVE('',#1467,#1460,#737,.T.);
#1824=EDGE_CURVE('',#1467,#1468,#738,.T.);
#1825=EDGE_CURVE('',#1461,#1468,#739,.T.);
#1826=EDGE_CURVE('',#1467,#1469,#581,.T.);
#1827=EDGE_CURVE('',#1469,#1470,#740,.T.);
#1828=EDGE_CURVE('',#1468,#1470,#582,.T.);
#1829=EDGE_CURVE('',#1469,#1471,#741,.T.);
#1830=EDGE_CURVE('',#1471,#1472,#742,.T.);
#1831=EDGE_CURVE('',#1470,#1472,#743,.T.);
#1832=EDGE_CURVE('',#1473,#1471,#583,.T.);
#1833=EDGE_CURVE('',#1473,#1474,#744,.T.);
#1834=EDGE_CURVE('',#1472,#1474,#584,.T.);
#1835=EDGE_CURVE('',#1475,#1476,#745,.T.);
#1836=EDGE_CURVE('',#1475,#1477,#746,.T.);
#1837=EDGE_CURVE('',#1478,#1477,#747,.T.);
#1838=EDGE_CURVE('',#1476,#1478,#748,.T.);
#1839=EDGE_CURVE('',#1479,#1475,#585,.T.);
#1840=EDGE_CURVE('',#1479,#1480,#749,.T.);
#1841=EDGE_CURVE('',#1477,#1480,#586,.T.);
#1842=EDGE_CURVE('',#1465,#1481,#750,.T.);
#1843=EDGE_CURVE('',#1482,#1481,#587,.T.);
#1844=EDGE_CURVE('',#1466,#1482,#751,.T.);
#1845=EDGE_CURVE('',#1483,#1484,#752,.T.);
#1846=EDGE_CURVE('',#1485,#1483,#753,.T.);
#1847=EDGE_CURVE('',#1485,#1486,#754,.T.);
#1848=EDGE_CURVE('',#1484,#1486,#755,.T.);
#1849=EDGE_CURVE('',#1487,#1488,#756,.T.);
#1850=EDGE_CURVE('',#1487,#1489,#757,.T.);
#1851=EDGE_CURVE('',#1489,#1490,#758,.T.);
#1852=EDGE_CURVE('',#1488,#1490,#759,.T.);
#1853=EDGE_CURVE('',#1491,#1492,#760,.T.);
#1854=EDGE_CURVE('',#1492,#1493,#761,.T.);
#1855=EDGE_CURVE('',#1494,#1493,#762,.T.);
#1856=EDGE_CURVE('',#1494,#1495,#763,.T.);
#1857=EDGE_CURVE('',#1495,#1496,#764,.T.);
#1858=EDGE_CURVE('',#1496,#1491,#765,.T.);
#1859=EDGE_CURVE('',#1497,#1498,#766,.T.);
#1860=EDGE_CURVE('',#1498,#1499,#767,.T.);
#1861=EDGE_CURVE('',#1499,#1500,#768,.T.);
#1862=EDGE_CURVE('',#1500,#1501,#769,.T.);
#1863=EDGE_CURVE('',#1502,#1501,#770,.T.);
#1864=EDGE_CURVE('',#1502,#1497,#771,.T.);
#1865=EDGE_CURVE('',#1464,#1457,#772,.T.);
#1866=EDGE_CURVE('',#1462,#1456,#773,.T.);
#1867=EDGE_CURVE('',#1503,#1473,#588,.T.);
#1868=EDGE_CURVE('',#1503,#1504,#774,.T.);
#1869=EDGE_CURVE('',#1474,#1504,#589,.T.);
#1870=EDGE_CURVE('',#1505,#1503,#775,.T.);
#1871=EDGE_CURVE('',#1505,#1506,#776,.T.);
#1872=EDGE_CURVE('',#1504,#1506,#777,.T.);
#1873=EDGE_CURVE('',#1507,#1505,#590,.T.);
#1874=EDGE_CURVE('',#1507,#1508,#778,.T.);
#1875=EDGE_CURVE('',#1509,#1508,#591,.T.);
#1876=EDGE_CURVE('',#1506,#1509,#779,.T.);
#1877=EDGE_CURVE('',#1493,#1510,#780,.T.);
#1878=EDGE_CURVE('',#1510,#1511,#781,.T.);
#1879=EDGE_CURVE('',#1511,#1512,#782,.T.);
#1880=EDGE_CURVE('',#1508,#1512,#783,.T.);
#1881=EDGE_CURVE('',#1507,#1463,#784,.T.);
#1882=EDGE_CURVE('',#1488,#1482,#785,.T.);
#1883=EDGE_CURVE('',#1490,#1493,#786,.T.);
#1884=EDGE_CURVE('',#1513,#1514,#592,.T.);
#1885=EDGE_CURVE('',#1513,#1515,#787,.T.);
#1886=EDGE_CURVE('',#1516,#1515,#593,.T.);
#1887=EDGE_CURVE('',#1514,#1516,#788,.T.);
#1888=EDGE_CURVE('',#1517,#1513,#789,.T.);
#1889=EDGE_CURVE('',#1517,#1518,#790,.T.);
#1890=EDGE_CURVE('',#1515,#1518,#791,.T.);
#1891=EDGE_CURVE('',#1506,#1516,#792,.T.);
#1892=EDGE_CURVE('',#1518,#1478,#594,.T.);
#1893=EDGE_CURVE('',#1480,#1465,#793,.T.);
#1894=EDGE_CURVE('',#1519,#1519,#595,.T.);
#1895=EDGE_CURVE('',#1519,#1520,#794,.T.);
#1896=EDGE_CURVE('',#1520,#1520,#596,.T.);
#1897=EDGE_CURVE('',#1521,#1522,#795,.T.);
#1898=EDGE_CURVE('',#1521,#1523,#796,.T.);
#1899=EDGE_CURVE('',#1523,#1524,#797,.T.);
#1900=EDGE_CURVE('',#1522,#1524,#798,.T.);
#1901=EDGE_CURVE('',#1525,#1489,#799,.T.);
#1902=EDGE_CURVE('',#1511,#1525,#800,.T.);
#1903=EDGE_CURVE('',#1510,#1526,#801,.T.);
#1904=EDGE_CURVE('',#1526,#1494,#802,.T.);
#1905=EDGE_CURVE('',#1512,#1527,#803,.T.);
#1906=EDGE_CURVE('',#1527,#1525,#804,.T.);
#1907=EDGE_CURVE('',#1527,#1487,#805,.T.);
#1908=EDGE_CURVE('',#1491,#1528,#806,.T.);
#1909=EDGE_CURVE('',#1529,#1528,#807,.T.);
#1910=EDGE_CURVE('',#1529,#1492,#808,.T.);
#1911=EDGE_CURVE('',#1510,#1529,#809,.T.);
#1912=EDGE_CURVE('',#1530,#1526,#810,.T.);
#1913=EDGE_CURVE('',#1530,#1495,#811,.T.);
#1914=EDGE_CURVE('',#1531,#1530,#812,.T.);
#1915=EDGE_CURVE('',#1531,#1496,#813,.T.);
#1916=EDGE_CURVE('',#1528,#1531,#814,.T.);
#1917=EDGE_CURVE('',#1532,#1533,#815,.T.);
#1918=EDGE_CURVE('',#1533,#1534,#816,.T.);
#1919=EDGE_CURVE('',#1535,#1534,#817,.T.);
#1920=EDGE_CURVE('',#1535,#1536,#818,.T.);
#1921=EDGE_CURVE('',#1536,#1537,#819,.T.);
#1922=EDGE_CURVE('',#1537,#1532,#820,.T.);
#1923=EDGE_CURVE('',#1476,#1517,#597,.T.);
#1924=EDGE_CURVE('',#1514,#1479,#821,.T.);
#1925=EDGE_CURVE('',#1522,#1509,#822,.T.);
#1926=EDGE_CURVE('',#1524,#1534,#823,.T.);
#1927=EDGE_CURVE('',#1534,#1502,#824,.T.);
#1928=EDGE_CURVE('',#1502,#1485,#825,.T.);
#1929=EDGE_CURVE('',#1481,#1483,#826,.T.);
#1930=EDGE_CURVE('',#1497,#1533,#827,.T.);
#1931=EDGE_CURVE('',#1532,#1498,#828,.T.);
#1932=EDGE_CURVE('',#1537,#1499,#829,.T.);
#1933=EDGE_CURVE('',#1536,#1500,#830,.T.);
#1934=EDGE_CURVE('',#1501,#1535,#831,.T.);
#1935=EDGE_CURVE('',#1486,#1523,#832,.T.);
#1936=EDGE_CURVE('',#1484,#1521,#833,.T.);
#2190=ORIENTED_EDGE('',*,*,#1705,.F.);
#2191=ORIENTED_EDGE('',*,*,#1706,.F.);
#2192=ORIENTED_EDGE('',*,*,#1707,.F.);
#2193=ORIENTED_EDGE('',*,*,#1708,.T.);
#2194=ORIENTED_EDGE('',*,*,#1709,.F.);
#2195=ORIENTED_EDGE('',*,*,#1706,.T.);
#2196=ORIENTED_EDGE('',*,*,#1710,.F.);
#2197=ORIENTED_EDGE('',*,*,#1708,.F.);
#2198=ORIENTED_EDGE('',*,*,#1711,.F.);
#2199=ORIENTED_EDGE('',*,*,#1712,.T.);
#2200=ORIENTED_EDGE('',*,*,#1713,.F.);
#2201=ORIENTED_EDGE('',*,*,#1712,.F.);
#2202=ORIENTED_EDGE('',*,*,#1714,.F.);
#2203=ORIENTED_EDGE('',*,*,#1715,.F.);
#2204=ORIENTED_EDGE('',*,*,#1716,.F.);
#2205=ORIENTED_EDGE('',*,*,#1717,.T.);
#2206=ORIENTED_EDGE('',*,*,#1718,.F.);
#2207=ORIENTED_EDGE('',*,*,#1717,.F.);
#2208=ORIENTED_EDGE('',*,*,#1714,.T.);
#2209=ORIENTED_EDGE('',*,*,#1716,.T.);
#2210=ORIENTED_EDGE('',*,*,#1719,.T.);
#2211=ORIENTED_EDGE('',*,*,#1720,.T.);
#2212=ORIENTED_EDGE('',*,*,#1721,.F.);
#2213=ORIENTED_EDGE('',*,*,#1722,.F.);
#2214=ORIENTED_EDGE('',*,*,#1723,.T.);
#2215=ORIENTED_EDGE('',*,*,#1724,.F.);
#2216=ORIENTED_EDGE('',*,*,#1725,.T.);
#2217=ORIENTED_EDGE('',*,*,#1726,.T.);
#2218=ORIENTED_EDGE('',*,*,#1725,.F.);
#2219=ORIENTED_EDGE('',*,*,#1726,.F.);
#2220=ORIENTED_EDGE('',*,*,#1727,.F.);
#2221=ORIENTED_EDGE('',*,*,#1728,.T.);
#2222=ORIENTED_EDGE('',*,*,#1729,.T.);
#2223=ORIENTED_EDGE('',*,*,#1728,.F.);
#2224=ORIENTED_EDGE('',*,*,#1729,.F.);
#2225=ORIENTED_EDGE('',*,*,#1730,.F.);
#2226=ORIENTED_EDGE('',*,*,#1720,.F.);
#2227=ORIENTED_EDGE('',*,*,#1731,.F.);
#2228=ORIENTED_EDGE('',*,*,#1732,.F.);
#2229=ORIENTED_EDGE('',*,*,#1733,.F.);
#2230=ORIENTED_EDGE('',*,*,#1734,.F.);
#2231=ORIENTED_EDGE('',*,*,#1735,.F.);
#2232=ORIENTED_EDGE('',*,*,#1736,.F.);
#2233=ORIENTED_EDGE('',*,*,#1737,.F.);
#2234=ORIENTED_EDGE('',*,*,#1738,.F.);
#2235=ORIENTED_EDGE('',*,*,#1739,.F.);
#2236=ORIENTED_EDGE('',*,*,#1740,.T.);
#2237=ORIENTED_EDGE('',*,*,#1736,.T.);
#2238=ORIENTED_EDGE('',*,*,#1741,.F.);
#2239=ORIENTED_EDGE('',*,*,#1742,.F.);
#2240=ORIENTED_EDGE('',*,*,#1743,.F.);
#2241=ORIENTED_EDGE('',*,*,#1744,.T.);
#2242=ORIENTED_EDGE('',*,*,#1745,.T.);
#2243=ORIENTED_EDGE('',*,*,#1745,.F.);
#2244=ORIENTED_EDGE('',*,*,#1746,.T.);
#2245=ORIENTED_EDGE('',*,*,#1747,.F.);
#2246=ORIENTED_EDGE('',*,*,#1746,.F.);
#2247=ORIENTED_EDGE('',*,*,#1734,.T.);
#2248=ORIENTED_EDGE('',*,*,#1748,.F.);
#2249=ORIENTED_EDGE('',*,*,#1749,.T.);
#2250=ORIENTED_EDGE('',*,*,#1750,.F.);
#2251=ORIENTED_EDGE('',*,*,#1751,.T.);
#2252=ORIENTED_EDGE('',*,*,#1752,.F.);
#2253=ORIENTED_EDGE('',*,*,#1753,.F.);
#2254=ORIENTED_EDGE('',*,*,#1754,.T.);
#2255=ORIENTED_EDGE('',*,*,#1755,.F.);
#2256=ORIENTED_EDGE('',*,*,#1756,.F.);
#2257=ORIENTED_EDGE('',*,*,#1757,.F.);
#2258=ORIENTED_EDGE('',*,*,#1756,.T.);
#2259=ORIENTED_EDGE('',*,*,#1758,.F.);
#2260=ORIENTED_EDGE('',*,*,#1749,.F.);
#2261=ORIENTED_EDGE('',*,*,#1759,.F.);
#2262=ORIENTED_EDGE('',*,*,#1743,.T.);
#2263=ORIENTED_EDGE('',*,*,#1742,.T.);
#2264=ORIENTED_EDGE('',*,*,#1760,.F.);
#2265=ORIENTED_EDGE('',*,*,#1751,.F.);
#2266=ORIENTED_EDGE('',*,*,#1761,.F.);
#2267=ORIENTED_EDGE('',*,*,#1762,.T.);
#2268=ORIENTED_EDGE('',*,*,#1761,.T.);
#2269=ORIENTED_EDGE('',*,*,#1763,.F.);
#2270=ORIENTED_EDGE('',*,*,#1764,.F.);
#2271=ORIENTED_EDGE('',*,*,#1765,.F.);
#2272=ORIENTED_EDGE('',*,*,#1766,.T.);
#2273=ORIENTED_EDGE('',*,*,#1767,.T.);
#2274=ORIENTED_EDGE('',*,*,#1738,.T.);
#2275=ORIENTED_EDGE('',*,*,#1767,.F.);
#2276=ORIENTED_EDGE('',*,*,#1768,.T.);
#2277=ORIENTED_EDGE('',*,*,#1769,.F.);
#2278=ORIENTED_EDGE('',*,*,#1739,.T.);
#2279=ORIENTED_EDGE('',*,*,#1715,.T.);
#2280=ORIENTED_EDGE('',*,*,#1723,.F.);
#2281=ORIENTED_EDGE('',*,*,#1770,.T.);
#2282=ORIENTED_EDGE('',*,*,#1771,.T.);
#2283=ORIENTED_EDGE('',*,*,#1731,.T.);
#2284=ORIENTED_EDGE('',*,*,#1719,.F.);
#2285=ORIENTED_EDGE('',*,*,#1771,.F.);
#2286=ORIENTED_EDGE('',*,*,#1772,.T.);
#2287=ORIENTED_EDGE('',*,*,#1773,.F.);
#2288=ORIENTED_EDGE('',*,*,#1732,.T.);
#2289=ORIENTED_EDGE('',*,*,#1774,.T.);
#2290=ORIENTED_EDGE('',*,*,#1775,.T.);
#2291=ORIENTED_EDGE('',*,*,#1776,.T.);
#2292=ORIENTED_EDGE('',*,*,#1777,.T.);
#2293=ORIENTED_EDGE('',*,*,#1778,.T.);
#2294=ORIENTED_EDGE('',*,*,#1779,.T.);
#2295=ORIENTED_EDGE('',*,*,#1721,.T.);
#2296=ORIENTED_EDGE('',*,*,#1730,.T.);
#2297=ORIENTED_EDGE('',*,*,#1752,.T.);
#2298=ORIENTED_EDGE('',*,*,#1760,.T.);
#2299=ORIENTED_EDGE('',*,*,#1741,.T.);
#2300=ORIENTED_EDGE('',*,*,#1735,.T.);
#2301=ORIENTED_EDGE('',*,*,#1747,.T.);
#2302=ORIENTED_EDGE('',*,*,#1727,.T.);
#2303=ORIENTED_EDGE('',*,*,#1780,.F.);
#2304=ORIENTED_EDGE('',*,*,#1781,.F.);
#2305=ORIENTED_EDGE('',*,*,#1782,.F.);
#2306=ORIENTED_EDGE('',*,*,#1764,.T.);
#2307=ORIENTED_EDGE('',*,*,#1779,.F.);
#2308=ORIENTED_EDGE('',*,*,#1783,.F.);
#2309=ORIENTED_EDGE('',*,*,#1784,.F.);
#2310=ORIENTED_EDGE('',*,*,#1772,.F.);
#2311=ORIENTED_EDGE('',*,*,#1770,.F.);
#2312=ORIENTED_EDGE('',*,*,#1722,.T.);
#2313=ORIENTED_EDGE('',*,*,#1769,.T.);
#2314=ORIENTED_EDGE('',*,*,#1785,.T.);
#2315=ORIENTED_EDGE('',*,*,#1774,.F.);
#2316=ORIENTED_EDGE('',*,*,#1740,.F.);
#2317=ORIENTED_EDGE('',*,*,#1718,.T.);
#2318=ORIENTED_EDGE('',*,*,#1775,.F.);
#2319=ORIENTED_EDGE('',*,*,#1785,.F.);
#2320=ORIENTED_EDGE('',*,*,#1768,.F.);
#2321=ORIENTED_EDGE('',*,*,#1766,.F.);
#2322=ORIENTED_EDGE('',*,*,#1786,.F.);
#2323=ORIENTED_EDGE('',*,*,#1787,.F.);
#2324=ORIENTED_EDGE('',*,*,#1783,.T.);
#2325=ORIENTED_EDGE('',*,*,#1778,.F.);
#2326=ORIENTED_EDGE('',*,*,#1788,.F.);
#2327=ORIENTED_EDGE('',*,*,#1789,.F.);
#2328=ORIENTED_EDGE('',*,*,#1790,.F.);
#2329=ORIENTED_EDGE('',*,*,#1791,.F.);
#2330=ORIENTED_EDGE('',*,*,#1792,.F.);
#2331=ORIENTED_EDGE('',*,*,#1790,.T.);
#2332=ORIENTED_EDGE('',*,*,#1793,.F.);
#2333=ORIENTED_EDGE('',*,*,#1794,.F.);
#2334=ORIENTED_EDGE('',*,*,#1795,.F.);
#2335=ORIENTED_EDGE('',*,*,#1794,.T.);
#2336=ORIENTED_EDGE('',*,*,#1796,.F.);
#2337=ORIENTED_EDGE('',*,*,#1797,.F.);
#2338=ORIENTED_EDGE('',*,*,#1798,.F.);
#2339=ORIENTED_EDGE('',*,*,#1797,.T.);
#2340=ORIENTED_EDGE('',*,*,#1799,.F.);
#2341=ORIENTED_EDGE('',*,*,#1754,.F.);
#2342=ORIENTED_EDGE('',*,*,#1800,.F.);
#2343=ORIENTED_EDGE('',*,*,#1781,.T.);
#2344=ORIENTED_EDGE('',*,*,#1801,.F.);
#2345=ORIENTED_EDGE('',*,*,#1802,.F.);
#2346=ORIENTED_EDGE('',*,*,#1803,.F.);
#2347=ORIENTED_EDGE('',*,*,#1802,.T.);
#2348=ORIENTED_EDGE('',*,*,#1804,.F.);
#2349=ORIENTED_EDGE('',*,*,#1805,.F.);
#2350=ORIENTED_EDGE('',*,*,#1806,.T.);
#2351=ORIENTED_EDGE('',*,*,#1805,.T.);
#2352=ORIENTED_EDGE('',*,*,#1807,.F.);
#2353=ORIENTED_EDGE('',*,*,#1808,.F.);
#2354=ORIENTED_EDGE('',*,*,#1809,.T.);
#2355=ORIENTED_EDGE('',*,*,#1808,.T.);
#2356=ORIENTED_EDGE('',*,*,#1810,.F.);
#2357=ORIENTED_EDGE('',*,*,#1811,.T.);
#2358=ORIENTED_EDGE('',*,*,#1787,.T.);
#2359=ORIENTED_EDGE('',*,*,#1812,.T.);
#2360=ORIENTED_EDGE('',*,*,#1813,.T.);
#2361=ORIENTED_EDGE('',*,*,#1814,.T.);
#2362=ORIENTED_EDGE('',*,*,#1776,.F.);
#2363=ORIENTED_EDGE('',*,*,#1815,.F.);
#2364=ORIENTED_EDGE('',*,*,#1816,.T.);
#2365=ORIENTED_EDGE('',*,*,#1817,.F.);
#2366=ORIENTED_EDGE('',*,*,#1788,.T.);
#2367=ORIENTED_EDGE('',*,*,#1777,.F.);
#2368=ORIENTED_EDGE('',*,*,#1814,.F.);
#2369=ORIENTED_EDGE('',*,*,#1813,.F.);
#2370=ORIENTED_EDGE('',*,*,#1818,.F.);
#2371=ORIENTED_EDGE('',*,*,#1819,.T.);
#2372=ORIENTED_EDGE('',*,*,#1820,.F.);
#2373=ORIENTED_EDGE('',*,*,#1821,.F.);
#2374=ORIENTED_EDGE('',*,*,#1822,.F.);
#2375=ORIENTED_EDGE('',*,*,#1823,.F.);
#2376=ORIENTED_EDGE('',*,*,#1824,.T.);
#2377=ORIENTED_EDGE('',*,*,#1825,.F.);
#2378=ORIENTED_EDGE('',*,*,#1816,.F.);
#2379=ORIENTED_EDGE('',*,*,#1826,.T.);
#2380=ORIENTED_EDGE('',*,*,#1827,.T.);
#2381=ORIENTED_EDGE('',*,*,#1828,.F.);
#2382=ORIENTED_EDGE('',*,*,#1824,.F.);
#2383=ORIENTED_EDGE('',*,*,#1829,.T.);
#2384=ORIENTED_EDGE('',*,*,#1830,.T.);
#2385=ORIENTED_EDGE('',*,*,#1831,.F.);
#2386=ORIENTED_EDGE('',*,*,#1827,.F.);
#2387=ORIENTED_EDGE('',*,*,#1832,.F.);
#2388=ORIENTED_EDGE('',*,*,#1833,.T.);
#2389=ORIENTED_EDGE('',*,*,#1834,.F.);
#2390=ORIENTED_EDGE('',*,*,#1830,.F.);
#2391=ORIENTED_EDGE('',*,*,#1835,.F.);
#2392=ORIENTED_EDGE('',*,*,#1836,.T.);
#2393=ORIENTED_EDGE('',*,*,#1837,.F.);
#2394=ORIENTED_EDGE('',*,*,#1838,.F.);
#2395=ORIENTED_EDGE('',*,*,#1839,.F.);
#2396=ORIENTED_EDGE('',*,*,#1840,.T.);
#2397=ORIENTED_EDGE('',*,*,#1841,.F.);
#2398=ORIENTED_EDGE('',*,*,#1836,.F.);
#2399=ORIENTED_EDGE('',*,*,#1821,.T.);
#2400=ORIENTED_EDGE('',*,*,#1842,.T.);
#2401=ORIENTED_EDGE('',*,*,#1843,.F.);
#2402=ORIENTED_EDGE('',*,*,#1844,.F.);
#2403=ORIENTED_EDGE('',*,*,#1845,.F.);
#2404=ORIENTED_EDGE('',*,*,#1846,.F.);
#2405=ORIENTED_EDGE('',*,*,#1847,.T.);
#2406=ORIENTED_EDGE('',*,*,#1848,.F.);
#2407=ORIENTED_EDGE('',*,*,#1849,.F.);
#2408=ORIENTED_EDGE('',*,*,#1850,.T.);
#2409=ORIENTED_EDGE('',*,*,#1851,.T.);
#2410=ORIENTED_EDGE('',*,*,#1852,.F.);
#2411=ORIENTED_EDGE('',*,*,#1853,.T.);
#2412=ORIENTED_EDGE('',*,*,#1854,.T.);
#2413=ORIENTED_EDGE('',*,*,#1855,.F.);
#2414=ORIENTED_EDGE('',*,*,#1856,.T.);
#2415=ORIENTED_EDGE('',*,*,#1857,.T.);
#2416=ORIENTED_EDGE('',*,*,#1858,.T.);
#2417=ORIENTED_EDGE('',*,*,#1859,.T.);
#2418=ORIENTED_EDGE('',*,*,#1860,.T.);
#2419=ORIENTED_EDGE('',*,*,#1861,.T.);
#2420=ORIENTED_EDGE('',*,*,#1862,.T.);
#2421=ORIENTED_EDGE('',*,*,#1863,.F.);
#2422=ORIENTED_EDGE('',*,*,#1864,.T.);
#2423=ORIENTED_EDGE('',*,*,#1865,.F.);
#2424=ORIENTED_EDGE('',*,*,#1819,.F.);
#2425=ORIENTED_EDGE('',*,*,#1866,.T.);
#2426=ORIENTED_EDGE('',*,*,#1811,.F.);
#2427=ORIENTED_EDGE('',*,*,#1867,.F.);
#2428=ORIENTED_EDGE('',*,*,#1868,.T.);
#2429=ORIENTED_EDGE('',*,*,#1869,.F.);
#2430=ORIENTED_EDGE('',*,*,#1833,.F.);
#2431=ORIENTED_EDGE('',*,*,#1870,.F.);
#2432=ORIENTED_EDGE('',*,*,#1871,.T.);
#2433=ORIENTED_EDGE('',*,*,#1872,.F.);
#2434=ORIENTED_EDGE('',*,*,#1868,.F.);
#2435=ORIENTED_EDGE('',*,*,#1873,.F.);
#2436=ORIENTED_EDGE('',*,*,#1874,.T.);
#2437=ORIENTED_EDGE('',*,*,#1875,.F.);
#2438=ORIENTED_EDGE('',*,*,#1876,.F.);
#2439=ORIENTED_EDGE('',*,*,#1871,.F.);
#2440=ORIENTED_EDGE('',*,*,#1877,.T.);
#2441=ORIENTED_EDGE('',*,*,#1878,.T.);
#2442=ORIENTED_EDGE('',*,*,#1879,.T.);
#2443=ORIENTED_EDGE('',*,*,#1880,.F.);
#2444=ORIENTED_EDGE('',*,*,#1874,.F.);
#2445=ORIENTED_EDGE('',*,*,#1881,.T.);
#2446=ORIENTED_EDGE('',*,*,#1822,.T.);
#2447=ORIENTED_EDGE('',*,*,#1844,.T.);
#2448=ORIENTED_EDGE('',*,*,#1882,.F.);
#2449=ORIENTED_EDGE('',*,*,#1852,.T.);
#2450=ORIENTED_EDGE('',*,*,#1883,.T.);
#2451=ORIENTED_EDGE('',*,*,#1884,.F.);
#2452=ORIENTED_EDGE('',*,*,#1885,.T.);
#2453=ORIENTED_EDGE('',*,*,#1886,.F.);
#2454=ORIENTED_EDGE('',*,*,#1887,.F.);
#2455=ORIENTED_EDGE('',*,*,#1888,.F.);
#2456=ORIENTED_EDGE('',*,*,#1889,.T.);
#2457=ORIENTED_EDGE('',*,*,#1890,.F.);
#2458=ORIENTED_EDGE('',*,*,#1885,.F.);
#2459=ORIENTED_EDGE('',*,*,#1869,.T.);
#2460=ORIENTED_EDGE('',*,*,#1872,.T.);
#2461=ORIENTED_EDGE('',*,*,#1891,.T.);
#2462=ORIENTED_EDGE('',*,*,#1886,.T.);
#2463=ORIENTED_EDGE('',*,*,#1890,.T.);
#2464=ORIENTED_EDGE('',*,*,#1892,.T.);
#2465=ORIENTED_EDGE('',*,*,#1837,.T.);
#2466=ORIENTED_EDGE('',*,*,#1841,.T.);
#2467=ORIENTED_EDGE('',*,*,#1893,.T.);
#2468=ORIENTED_EDGE('',*,*,#1820,.T.);
#2469=ORIENTED_EDGE('',*,*,#1865,.T.);
#2470=ORIENTED_EDGE('',*,*,#1810,.T.);
#2471=ORIENTED_EDGE('',*,*,#1807,.T.);
#2472=ORIENTED_EDGE('',*,*,#1804,.T.);
#2473=ORIENTED_EDGE('',*,*,#1801,.T.);
#2474=ORIENTED_EDGE('',*,*,#1780,.T.);
#2475=ORIENTED_EDGE('',*,*,#1763,.T.);
#2476=ORIENTED_EDGE('',*,*,#1750,.T.);
#2477=ORIENTED_EDGE('',*,*,#1758,.T.);
#2478=ORIENTED_EDGE('',*,*,#1755,.T.);
#2479=ORIENTED_EDGE('',*,*,#1799,.T.);
#2480=ORIENTED_EDGE('',*,*,#1796,.T.);
#2481=ORIENTED_EDGE('',*,*,#1793,.T.);
#2482=ORIENTED_EDGE('',*,*,#1789,.T.);
#2483=ORIENTED_EDGE('',*,*,#1817,.T.);
#2484=ORIENTED_EDGE('',*,*,#1825,.T.);
#2485=ORIENTED_EDGE('',*,*,#1828,.T.);
#2486=ORIENTED_EDGE('',*,*,#1831,.T.);
#2487=ORIENTED_EDGE('',*,*,#1834,.T.);
#2488=ORIENTED_EDGE('',*,*,#1894,.F.);
#2489=ORIENTED_EDGE('',*,*,#1895,.T.);
#2490=ORIENTED_EDGE('',*,*,#1896,.F.);
#2491=ORIENTED_EDGE('',*,*,#1895,.F.);
#2492=ORIENTED_EDGE('',*,*,#1894,.T.);
#2493=ORIENTED_EDGE('',*,*,#1897,.F.);
#2494=ORIENTED_EDGE('',*,*,#1898,.T.);
#2495=ORIENTED_EDGE('',*,*,#1899,.T.);
#2496=ORIENTED_EDGE('',*,*,#1900,.F.);
#2497=ORIENTED_EDGE('',*,*,#1901,.F.);
#2498=ORIENTED_EDGE('',*,*,#1902,.F.);
#2499=ORIENTED_EDGE('',*,*,#1878,.F.);
#2500=ORIENTED_EDGE('',*,*,#1903,.T.);
#2501=ORIENTED_EDGE('',*,*,#1904,.T.);
#2502=ORIENTED_EDGE('',*,*,#1855,.T.);
#2503=ORIENTED_EDGE('',*,*,#1883,.F.);
#2504=ORIENTED_EDGE('',*,*,#1851,.F.);
#2505=ORIENTED_EDGE('',*,*,#1905,.F.);
#2506=ORIENTED_EDGE('',*,*,#1879,.F.);
#2507=ORIENTED_EDGE('',*,*,#1902,.T.);
#2508=ORIENTED_EDGE('',*,*,#1906,.F.);
#2509=ORIENTED_EDGE('',*,*,#1907,.F.);
#2510=ORIENTED_EDGE('',*,*,#1906,.T.);
#2511=ORIENTED_EDGE('',*,*,#1901,.T.);
#2512=ORIENTED_EDGE('',*,*,#1850,.F.);
#2513=ORIENTED_EDGE('',*,*,#1908,.T.);
#2514=ORIENTED_EDGE('',*,*,#1909,.F.);
#2515=ORIENTED_EDGE('',*,*,#1910,.T.);
#2516=ORIENTED_EDGE('',*,*,#1853,.F.);
#2517=ORIENTED_EDGE('',*,*,#1910,.F.);
#2518=ORIENTED_EDGE('',*,*,#1911,.F.);
#2519=ORIENTED_EDGE('',*,*,#1877,.F.);
#2520=ORIENTED_EDGE('',*,*,#1854,.F.);
#2521=ORIENTED_EDGE('',*,*,#1711,.T.);
#2522=ORIENTED_EDGE('',*,*,#1904,.F.);
#2523=ORIENTED_EDGE('',*,*,#1912,.F.);
#2524=ORIENTED_EDGE('',*,*,#1913,.T.);
#2525=ORIENTED_EDGE('',*,*,#1856,.F.);
#2526=ORIENTED_EDGE('',*,*,#1713,.T.);
#2527=ORIENTED_EDGE('',*,*,#1913,.F.);
#2528=ORIENTED_EDGE('',*,*,#1914,.F.);
#2529=ORIENTED_EDGE('',*,*,#1915,.T.);
#2530=ORIENTED_EDGE('',*,*,#1857,.F.);
#2531=ORIENTED_EDGE('',*,*,#1915,.F.);
#2532=ORIENTED_EDGE('',*,*,#1916,.F.);
#2533=ORIENTED_EDGE('',*,*,#1908,.F.);
#2534=ORIENTED_EDGE('',*,*,#1858,.F.);
#2535=ORIENTED_EDGE('',*,*,#1909,.T.);
#2536=ORIENTED_EDGE('',*,*,#1916,.T.);
#2537=ORIENTED_EDGE('',*,*,#1914,.T.);
#2538=ORIENTED_EDGE('',*,*,#1912,.T.);
#2539=ORIENTED_EDGE('',*,*,#1903,.F.);
#2540=ORIENTED_EDGE('',*,*,#1911,.T.);
#2541=ORIENTED_EDGE('',*,*,#1917,.T.);
#2542=ORIENTED_EDGE('',*,*,#1918,.T.);
#2543=ORIENTED_EDGE('',*,*,#1919,.F.);
#2544=ORIENTED_EDGE('',*,*,#1920,.T.);
#2545=ORIENTED_EDGE('',*,*,#1921,.T.);
#2546=ORIENTED_EDGE('',*,*,#1922,.T.);
#2547=ORIENTED_EDGE('',*,*,#1765,.T.);
#2548=ORIENTED_EDGE('',*,*,#1737,.T.);
#2549=ORIENTED_EDGE('',*,*,#1744,.F.);
#2550=ORIENTED_EDGE('',*,*,#1759,.T.);
#2551=ORIENTED_EDGE('',*,*,#1762,.F.);
#2552=ORIENTED_EDGE('',*,*,#1782,.T.);
#2553=ORIENTED_EDGE('',*,*,#1800,.T.);
#2554=ORIENTED_EDGE('',*,*,#1803,.T.);
#2555=ORIENTED_EDGE('',*,*,#1806,.F.);
#2556=ORIENTED_EDGE('',*,*,#1809,.F.);
#2557=ORIENTED_EDGE('',*,*,#1866,.F.);
#2558=ORIENTED_EDGE('',*,*,#1818,.T.);
#2559=ORIENTED_EDGE('',*,*,#1881,.F.);
#2560=ORIENTED_EDGE('',*,*,#1873,.T.);
#2561=ORIENTED_EDGE('',*,*,#1870,.T.);
#2562=ORIENTED_EDGE('',*,*,#1867,.T.);
#2563=ORIENTED_EDGE('',*,*,#1832,.T.);
#2564=ORIENTED_EDGE('',*,*,#1829,.F.);
#2565=ORIENTED_EDGE('',*,*,#1826,.F.);
#2566=ORIENTED_EDGE('',*,*,#1823,.T.);
#2567=ORIENTED_EDGE('',*,*,#1815,.T.);
#2568=ORIENTED_EDGE('',*,*,#1812,.F.);
#2569=ORIENTED_EDGE('',*,*,#1786,.T.);
#2570=ORIENTED_EDGE('',*,*,#1773,.T.);
#2571=ORIENTED_EDGE('',*,*,#1784,.T.);
#2572=ORIENTED_EDGE('',*,*,#1791,.T.);
#2573=ORIENTED_EDGE('',*,*,#1792,.T.);
#2574=ORIENTED_EDGE('',*,*,#1795,.T.);
#2575=ORIENTED_EDGE('',*,*,#1798,.T.);
#2576=ORIENTED_EDGE('',*,*,#1753,.T.);
#2577=ORIENTED_EDGE('',*,*,#1757,.T.);
#2578=ORIENTED_EDGE('',*,*,#1748,.T.);
#2579=ORIENTED_EDGE('',*,*,#1733,.T.);
#2580=ORIENTED_EDGE('',*,*,#1923,.T.);
#2581=ORIENTED_EDGE('',*,*,#1888,.T.);
#2582=ORIENTED_EDGE('',*,*,#1884,.T.);
#2583=ORIENTED_EDGE('',*,*,#1924,.T.);
#2584=ORIENTED_EDGE('',*,*,#1839,.T.);
#2585=ORIENTED_EDGE('',*,*,#1835,.T.);
#2586=ORIENTED_EDGE('',*,*,#1892,.F.);
#2587=ORIENTED_EDGE('',*,*,#1889,.F.);
#2588=ORIENTED_EDGE('',*,*,#1923,.F.);
#2589=ORIENTED_EDGE('',*,*,#1838,.T.);
#2590=ORIENTED_EDGE('',*,*,#1924,.F.);
#2591=ORIENTED_EDGE('',*,*,#1887,.T.);
#2592=ORIENTED_EDGE('',*,*,#1891,.F.);
#2593=ORIENTED_EDGE('',*,*,#1876,.T.);
#2594=ORIENTED_EDGE('',*,*,#1925,.F.);
#2595=ORIENTED_EDGE('',*,*,#1900,.T.);
#2596=ORIENTED_EDGE('',*,*,#1926,.T.);
#2597=ORIENTED_EDGE('',*,*,#1927,.T.);
#2598=ORIENTED_EDGE('',*,*,#1928,.T.);
#2599=ORIENTED_EDGE('',*,*,#1846,.T.);
#2600=ORIENTED_EDGE('',*,*,#1929,.F.);
#2601=ORIENTED_EDGE('',*,*,#1842,.F.);
#2602=ORIENTED_EDGE('',*,*,#1893,.F.);
#2603=ORIENTED_EDGE('',*,*,#1840,.F.);
#2604=ORIENTED_EDGE('',*,*,#1927,.F.);
#2605=ORIENTED_EDGE('',*,*,#1918,.F.);
#2606=ORIENTED_EDGE('',*,*,#1930,.F.);
#2607=ORIENTED_EDGE('',*,*,#1864,.F.);
#2608=ORIENTED_EDGE('',*,*,#1709,.T.);
#2609=ORIENTED_EDGE('',*,*,#1710,.T.);
#2610=ORIENTED_EDGE('',*,*,#1705,.T.);
#2611=ORIENTED_EDGE('',*,*,#1930,.T.);
#2612=ORIENTED_EDGE('',*,*,#1917,.F.);
#2613=ORIENTED_EDGE('',*,*,#1931,.T.);
#2614=ORIENTED_EDGE('',*,*,#1859,.F.);
#2615=ORIENTED_EDGE('',*,*,#1931,.F.);
#2616=ORIENTED_EDGE('',*,*,#1922,.F.);
#2617=ORIENTED_EDGE('',*,*,#1932,.T.);
#2618=ORIENTED_EDGE('',*,*,#1860,.F.);
#2619=ORIENTED_EDGE('',*,*,#1932,.F.);
#2620=ORIENTED_EDGE('',*,*,#1921,.F.);
#2621=ORIENTED_EDGE('',*,*,#1933,.T.);
#2622=ORIENTED_EDGE('',*,*,#1861,.F.);
#2623=ORIENTED_EDGE('',*,*,#1933,.F.);
#2624=ORIENTED_EDGE('',*,*,#1920,.F.);
#2625=ORIENTED_EDGE('',*,*,#1934,.F.);
#2626=ORIENTED_EDGE('',*,*,#1862,.F.);
#2627=ORIENTED_EDGE('',*,*,#1707,.T.);
#2628=ORIENTED_EDGE('',*,*,#1934,.T.);
#2629=ORIENTED_EDGE('',*,*,#1919,.T.);
#2630=ORIENTED_EDGE('',*,*,#1926,.F.);
#2631=ORIENTED_EDGE('',*,*,#1899,.F.);
#2632=ORIENTED_EDGE('',*,*,#1935,.F.);
#2633=ORIENTED_EDGE('',*,*,#1847,.F.);
#2634=ORIENTED_EDGE('',*,*,#1928,.F.);
#2635=ORIENTED_EDGE('',*,*,#1863,.T.);
#2636=ORIENTED_EDGE('',*,*,#1935,.T.);
#2637=ORIENTED_EDGE('',*,*,#1898,.F.);
#2638=ORIENTED_EDGE('',*,*,#1936,.F.);
#2639=ORIENTED_EDGE('',*,*,#1848,.T.);
#2640=ORIENTED_EDGE('',*,*,#1936,.T.);
#2641=ORIENTED_EDGE('',*,*,#1897,.T.);
#2642=ORIENTED_EDGE('',*,*,#1925,.T.);
#2643=ORIENTED_EDGE('',*,*,#1875,.T.);
#2644=ORIENTED_EDGE('',*,*,#1880,.T.);
#2645=ORIENTED_EDGE('',*,*,#1905,.T.);
#2646=ORIENTED_EDGE('',*,*,#1907,.T.);
#2647=ORIENTED_EDGE('',*,*,#1849,.T.);
#2648=ORIENTED_EDGE('',*,*,#1882,.T.);
#2649=ORIENTED_EDGE('',*,*,#1843,.T.);
#2650=ORIENTED_EDGE('',*,*,#1929,.T.);
#2651=ORIENTED_EDGE('',*,*,#1845,.T.);
#2652=ORIENTED_EDGE('',*,*,#1724,.T.);
#2653=ORIENTED_EDGE('',*,*,#1896,.T.);
#3160=PLANE('',#3569);
#3161=PLANE('',#3583);
#3162=PLANE('',#3587);
#3163=PLANE('',#3591);
#3164=PLANE('',#3592);
#3165=PLANE('',#3593);
#3166=PLANE('',#3594);
#3167=PLANE('',#3595);
#3168=PLANE('',#3599);
#3169=PLANE('',#3600);
#3170=PLANE('',#3607);
#3171=PLANE('',#3608);
#3172=PLANE('',#3609);
#3173=PLANE('',#3610);
#3174=PLANE('',#3611);
#3175=PLANE('',#3612);
#3176=PLANE('',#3617);
#3177=PLANE('',#3618);
#3178=PLANE('',#3619);
#3179=PLANE('',#3620);
#3180=PLANE('',#3624);
#3181=PLANE('',#3628);
#3182=PLANE('',#3632);
#3183=PLANE('',#3636);
#3184=PLANE('',#3644);
#3185=PLANE('',#3648);
#3186=PLANE('',#3652);
#3187=PLANE('',#3658);
#3188=PLANE('',#3659);
#3189=PLANE('',#3660);
#3190=PLANE('',#3661);
#3191=PLANE('',#3662);
#3192=PLANE('',#3666);
#3193=PLANE('',#3670);
#3194=PLANE('',#3674);
#3195=PLANE('',#3675);
#3196=PLANE('',#3680);
#3197=PLANE('',#3681);
#3198=PLANE('',#3682);
#3199=PLANE('',#3683);
#3200=PLANE('',#3684);
#3201=PLANE('',#3685);
#3202=PLANE('',#3686);
#3203=PLANE('',#3687);
#3204=PLANE('',#3688);
#3205=PLANE('',#3689);
#3206=PLANE('',#3690);
#3207=PLANE('',#3691);
#3208=PLANE('',#3692);
#3209=PLANE('',#3695);
#3210=PLANE('',#3696);
#3211=PLANE('',#3697);
#3212=PLANE('',#3698);
#3213=PLANE('',#3699);
#3214=PLANE('',#3700);
#3215=PLANE('',#3701);
#3216=PLANE('',#3702);
#3217=PLANE('',#3703);
#3288=ADVANCED_FACE('',(#168),#3160,.T.);
#3289=ADVANCED_FACE('',(#169),#114,.F.);
#3290=ADVANCED_FACE('',(#170),#115,.F.);
#3291=ADVANCED_FACE('',(#171),#116,.F.);
#3292=ADVANCED_FACE('',(#172),#3161,.F.);
#3293=ADVANCED_FACE('',(#173),#117,.F.);
#3294=ADVANCED_FACE('',(#174),#3162,.T.);
#3295=ADVANCED_FACE('',(#175),#118,.F.);
#3296=ADVANCED_FACE('',(#176),#3163,.T.);
#3297=ADVANCED_FACE('',(#177),#3164,.F.);
#3298=ADVANCED_FACE('',(#178),#3165,.F.);
#3299=ADVANCED_FACE('',(#179),#3166,.T.);
#3300=ADVANCED_FACE('',(#180),#3167,.F.);
#3301=ADVANCED_FACE('',(#181),#119,.F.);
#3302=ADVANCED_FACE('',(#182),#3168,.T.);
#3303=ADVANCED_FACE('',(#183),#3169,.T.);
#3304=ADVANCED_FACE('',(#184),#120,.F.);
#3305=ADVANCED_FACE('',(#185),#121,.T.);
#3306=ADVANCED_FACE('',(#186),#3170,.T.);
#3307=ADVANCED_FACE('',(#187),#3171,.F.);
#3308=ADVANCED_FACE('',(#188),#3172,.F.);
#3309=ADVANCED_FACE('',(#189),#3173,.F.);
#3310=ADVANCED_FACE('',(#190),#3174,.F.);
#3311=ADVANCED_FACE('',(#191,#75,#76),#3175,.F.);
#3312=ADVANCED_FACE('',(#192),#122,.T.);
#3313=ADVANCED_FACE('',(#193),#3176,.F.);
#3314=ADVANCED_FACE('',(#194,#77),#3177,.F.);
#3315=ADVANCED_FACE('',(#195),#3178,.F.);
#3316=ADVANCED_FACE('',(#196),#3179,.T.);
#3317=ADVANCED_FACE('',(#197),#123,.F.);
#3318=ADVANCED_FACE('',(#198),#3180,.T.);
#3319=ADVANCED_FACE('',(#199),#124,.F.);
#3320=ADVANCED_FACE('',(#200),#3181,.T.);
#3321=ADVANCED_FACE('',(#201),#125,.T.);
#3322=ADVANCED_FACE('',(#202),#3182,.T.);
#3323=ADVANCED_FACE('',(#203),#126,.F.);
#3324=ADVANCED_FACE('',(#204),#3183,.T.);
#3325=ADVANCED_FACE('',(#205),#127,.T.);
#3326=ADVANCED_FACE('',(#206),#128,.T.);
#3327=ADVANCED_FACE('',(#207),#3184,.T.);
#3328=ADVANCED_FACE('',(#208),#129,.F.);
#3329=ADVANCED_FACE('',(#209),#3185,.T.);
#3330=ADVANCED_FACE('',(#210),#130,.T.);
#3331=ADVANCED_FACE('',(#211),#3186,.T.);
#3332=ADVANCED_FACE('',(#212),#131,.F.);
#3333=ADVANCED_FACE('',(#213),#132,.T.);
#3334=ADVANCED_FACE('',(#214),#3187,.F.);
#3335=ADVANCED_FACE('',(#215),#3188,.F.);
#3336=ADVANCED_FACE('',(#216),#3189,.T.);
#3337=ADVANCED_FACE('',(#217),#3190,.T.);
#3338=ADVANCED_FACE('',(#218),#3191,.T.);
#3339=ADVANCED_FACE('',(#219),#133,.T.);
#3340=ADVANCED_FACE('',(#220),#3192,.T.);
#3341=ADVANCED_FACE('',(#221),#134,.T.);
#3342=ADVANCED_FACE('',(#222),#3193,.T.);
#3343=ADVANCED_FACE('',(#223),#135,.F.);
#3344=ADVANCED_FACE('',(#224),#3194,.T.);
#3345=ADVANCED_FACE('',(#225),#3195,.F.);
#3346=ADVANCED_FACE('',(#226),#136,.F.);
#3347=ADVANCED_FACE('',(#227),#3196,.F.);
#3348=ADVANCED_FACE('',(#228),#3197,.F.);
#3349=ADVANCED_FACE('',(#229),#3198,.F.);
#3350=ADVANCED_FACE('',(#230),#3199,.F.);
#3351=ADVANCED_FACE('',(#231),#3200,.F.);
#3352=ADVANCED_FACE('',(#232),#3201,.T.);
#3353=ADVANCED_FACE('',(#233,#78),#3202,.T.);
#3354=ADVANCED_FACE('',(#234,#79),#3203,.T.);
#3355=ADVANCED_FACE('',(#235),#3204,.T.);
#3356=ADVANCED_FACE('',(#236),#3205,.T.);
#3357=ADVANCED_FACE('',(#237),#3206,.T.);
#3358=ADVANCED_FACE('',(#238),#3207,.T.);
#3359=ADVANCED_FACE('',(#239,#80,#81),#3208,.T.);
#3360=ADVANCED_FACE('',(#240),#137,.F.);
#3361=ADVANCED_FACE('',(#241),#3209,.T.);
#3362=ADVANCED_FACE('',(#242,#82),#3210,.T.);
#3363=ADVANCED_FACE('',(#243),#3211,.T.);
#3364=ADVANCED_FACE('',(#244),#3212,.T.);
#3365=ADVANCED_FACE('',(#245),#3213,.T.);
#3366=ADVANCED_FACE('',(#246,#83),#3214,.T.);
#3367=ADVANCED_FACE('',(#247),#3215,.F.);
#3368=ADVANCED_FACE('',(#248),#3216,.F.);
#3369=ADVANCED_FACE('',(#249,#84,#85),#3217,.F.);
#3470=CLOSED_SHELL('',(#3288,#3289,#3290,#3291,#3292,#3293,#3294,#3295,
#3296,#3297,#3298,#3299,#3300,#3301,#3302,#3303,#3304,#3305,#3306,#3307,
#3308,#3309,#3310,#3311,#3312,#3313,#3314,#3315,#3316,#3317,#3318,#3319,
#3320,#3321,#3322,#3323,#3324,#3325,#3326,#3327,#3328,#3329,#3330,#3331,
#3332,#3333,#3334,#3335,#3336,#3337,#3338,#3339,#3340,#3341,#3342,#3343,
#3344,#3345,#3346,#3347,#3348,#3349,#3350,#3351,#3352,#3353,#3354,#3355,
#3356,#3357,#3358,#3359,#3360,#3361,#3362,#3363,#3364,#3365,#3366,#3367,
#3368,#3369));
#3568=AXIS2_PLACEMENT_3D('',#4890,#3888,#3889);
#3569=AXIS2_PLACEMENT_3D('',#4891,#3890,#3891);
#3570=AXIS2_PLACEMENT_3D('',#4895,#3893,#3894);
#3571=AXIS2_PLACEMENT_3D('',#4896,#3895,#3896);
#3572=AXIS2_PLACEMENT_3D('',#4898,#3897,#3898);
#3573=AXIS2_PLACEMENT_3D('',#4901,#3900,#3901);
#3574=AXIS2_PLACEMENT_3D('',#4902,#3902,#3903);
#3575=AXIS2_PLACEMENT_3D('',#4903,#3904,#3905);
#3576=AXIS2_PLACEMENT_3D('',#4905,#3906,#3907);
#3577=AXIS2_PLACEMENT_3D('',#4908,#3909,#3910);
#3578=AXIS2_PLACEMENT_3D('',#4909,#3911,#3912);
#3579=AXIS2_PLACEMENT_3D('',#4912,#3913,#3914);
#3580=AXIS2_PLACEMENT_3D('',#4914,#3915,#3916);
#3581=AXIS2_PLACEMENT_3D('',#4915,#3917,#3918);
#3582=AXIS2_PLACEMENT_3D('',#4918,#3920,#3921);
#3583=AXIS2_PLACEMENT_3D('',#4919,#3922,#3923);
#3584=AXIS2_PLACEMENT_3D('',#4929,#3929,#3930);
#3585=AXIS2_PLACEMENT_3D('',#4931,#3931,#3932);
#3586=AXIS2_PLACEMENT_3D('',#4934,#3934,#3935);
#3587=AXIS2_PLACEMENT_3D('',#4935,#3936,#3937);
#3588=AXIS2_PLACEMENT_3D('',#4936,#3938,#3939);
#3589=AXIS2_PLACEMENT_3D('',#4938,#3940,#3941);
#3590=AXIS2_PLACEMENT_3D('',#4941,#3943,#3944);
#3591=AXIS2_PLACEMENT_3D('',#4942,#3945,#3946);
#3592=AXIS2_PLACEMENT_3D('',#4943,#3947,#3948);
#3593=AXIS2_PLACEMENT_3D('',#4953,#3954,#3955);
#3594=AXIS2_PLACEMENT_3D('',#4966,#3962,#3963);
#3595=AXIS2_PLACEMENT_3D('',#4974,#3968,#3969);
#3596=AXIS2_PLACEMENT_3D('',#4976,#3970,#3971);
#3597=AXIS2_PLACEMENT_3D('',#4977,#3972,#3973);
#3598=AXIS2_PLACEMENT_3D('',#4980,#3975,#3976);
#3599=AXIS2_PLACEMENT_3D('',#4981,#3977,#3978);
#3600=AXIS2_PLACEMENT_3D('',#4991,#3984,#3985);
#3601=AXIS2_PLACEMENT_3D('',#5000,#3990,#3991);
#3602=AXIS2_PLACEMENT_3D('',#5001,#3992,#3993);
#3603=AXIS2_PLACEMENT_3D('',#5002,#3994,#3995);
#3604=AXIS2_PLACEMENT_3D('',#5003,#3996,#3997);
#3605=AXIS2_PLACEMENT_3D('',#5005,#3998,#3999);
#3606=AXIS2_PLACEMENT_3D('',#5006,#4000,#4001);
#3607=AXIS2_PLACEMENT_3D('',#5008,#4003,#4004);
#3608=AXIS2_PLACEMENT_3D('',#5014,#4008,#4009);
#3609=AXIS2_PLACEMENT_3D('',#5020,#4013,#4014);
#3610=AXIS2_PLACEMENT_3D('',#5024,#4017,#4018);
#3611=AXIS2_PLACEMENT_3D('',#5028,#4021,#4022);
#3612=AXIS2_PLACEMENT_3D('',#5032,#4025,#4026);
#3613=AXIS2_PLACEMENT_3D('',#5040,#4030,#4031);
#3614=AXIS2_PLACEMENT_3D('',#5044,#4034,#4035);
#3615=AXIS2_PLACEMENT_3D('',#5046,#4036,#4037);
#3616=AXIS2_PLACEMENT_3D('',#5049,#4039,#4040);
#3617=AXIS2_PLACEMENT_3D('',#5050,#4041,#4042);
#3618=AXIS2_PLACEMENT_3D('',#5054,#4045,#4046);
#3619=AXIS2_PLACEMENT_3D('',#5056,#4048,#4049);
#3620=AXIS2_PLACEMENT_3D('',#5060,#4052,#4053);
#3621=AXIS2_PLACEMENT_3D('',#5068,#4058,#4059);
#3622=AXIS2_PLACEMENT_3D('',#5070,#4060,#4061);
#3623=AXIS2_PLACEMENT_3D('',#5072,#4062,#4063);
#3624=AXIS2_PLACEMENT_3D('',#5074,#4065,#4066);
#3625=AXIS2_PLACEMENT_3D('',#5080,#4070,#4071);
#3626=AXIS2_PLACEMENT_3D('',#5081,#4072,#4073);
#3627=AXIS2_PLACEMENT_3D('',#5082,#4074,#4075);
#3628=AXIS2_PLACEMENT_3D('',#5083,#4076,#4077);
#3629=AXIS2_PLACEMENT_3D('',#5089,#4081,#4082);
#3630=AXIS2_PLACEMENT_3D('',#5091,#4083,#4084);
#3631=AXIS2_PLACEMENT_3D('',#5093,#4085,#4086);
#3632=AXIS2_PLACEMENT_3D('',#5095,#4088,#4089);
#3633=AXIS2_PLACEMENT_3D('',#5101,#4093,#4094);
#3634=AXIS2_PLACEMENT_3D('',#5103,#4095,#4096);
#3635=AXIS2_PLACEMENT_3D('',#5105,#4097,#4098);
#3636=AXIS2_PLACEMENT_3D('',#5107,#4100,#4101);
#3637=AXIS2_PLACEMENT_3D('',#5113,#4105,#4106);
#3638=AXIS2_PLACEMENT_3D('',#5115,#4107,#4108);
#3639=AXIS2_PLACEMENT_3D('',#5118,#4110,#4111);
#3640=AXIS2_PLACEMENT_3D('',#5119,#4112,#4113);
#3641=AXIS2_PLACEMENT_3D('',#5122,#4114,#4115);
#3642=AXIS2_PLACEMENT_3D('',#5126,#4117,#4118);
#3643=AXIS2_PLACEMENT_3D('',#5128,#4119,#4120);
#3644=AXIS2_PLACEMENT_3D('',#5130,#4122,#4123);
#3645=AXIS2_PLACEMENT_3D('',#5136,#4127,#4128);
#3646=AXIS2_PLACEMENT_3D('',#5138,#4129,#4130);
#3647=AXIS2_PLACEMENT_3D('',#5141,#4132,#4133);
#3648=AXIS2_PLACEMENT_3D('',#5142,#4134,#4135);
#3649=AXIS2_PLACEMENT_3D('',#5148,#4139,#4140);
#3650=AXIS2_PLACEMENT_3D('',#5150,#4141,#4142);
#3651=AXIS2_PLACEMENT_3D('',#5153,#4144,#4145);
#3652=AXIS2_PLACEMENT_3D('',#5154,#4146,#4147);
#3653=AXIS2_PLACEMENT_3D('',#5163,#4152,#4153);
#3654=AXIS2_PLACEMENT_3D('',#5165,#4154,#4155);
#3655=AXIS2_PLACEMENT_3D('',#5168,#4157,#4158);
#3656=AXIS2_PLACEMENT_3D('',#5169,#4159,#4160);
#3657=AXIS2_PLACEMENT_3D('',#5173,#4162,#4163);
#3658=AXIS2_PLACEMENT_3D('',#5175,#4165,#4166);
#3659=AXIS2_PLACEMENT_3D('',#5184,#4171,#4172);
#3660=AXIS2_PLACEMENT_3D('',#5193,#4177,#4178);
#3661=AXIS2_PLACEMENT_3D('',#5206,#4185,#4186);
#3662=AXIS2_PLACEMENT_3D('',#5219,#4193,#4194);
#3663=AXIS2_PLACEMENT_3D('',#5222,#4197,#4198);
#3664=AXIS2_PLACEMENT_3D('',#5224,#4199,#4200);
#3665=AXIS2_PLACEMENT_3D('',#5227,#4202,#4203);
#3666=AXIS2_PLACEMENT_3D('',#5228,#4204,#4205);
#3667=AXIS2_PLACEMENT_3D('',#5234,#4209,#4210);
#3668=AXIS2_PLACEMENT_3D('',#5236,#4211,#4212);
#3669=AXIS2_PLACEMENT_3D('',#5240,#4214,#4215);
#3670=AXIS2_PLACEMENT_3D('',#5242,#4217,#4218);
#3671=AXIS2_PLACEMENT_3D('',#5253,#4226,#4227);
#3672=AXIS2_PLACEMENT_3D('',#5256,#4228,#4229);
#3673=AXIS2_PLACEMENT_3D('',#5260,#4231,#4232);
#3674=AXIS2_PLACEMENT_3D('',#5262,#4234,#4235);
#3675=AXIS2_PLACEMENT_3D('',#5268,#4239,#4240);
#3676=AXIS2_PLACEMENT_3D('',#5270,#4242,#4243);
#3677=AXIS2_PLACEMENT_3D('',#5272,#4245,#4246);
#3678=AXIS2_PLACEMENT_3D('',#5274,#4247,#4248);
#3679=AXIS2_PLACEMENT_3D('',#5277,#4250,#4251);
#3680=AXIS2_PLACEMENT_3D('',#5278,#4252,#4253);
#3681=AXIS2_PLACEMENT_3D('',#5279,#4254,#4255);
#3682=AXIS2_PLACEMENT_3D('',#5288,#4260,#4261);
#3683=AXIS2_PLACEMENT_3D('',#5295,#4266,#4267);
#3684=AXIS2_PLACEMENT_3D('',#5299,#4270,#4271);
#3685=AXIS2_PLACEMENT_3D('',#5301,#4273,#4274);
#3686=AXIS2_PLACEMENT_3D('',#5307,#4278,#4279);
#3687=AXIS2_PLACEMENT_3D('',#5309,#4281,#4282);
#3688=AXIS2_PLACEMENT_3D('',#5313,#4285,#4286);
#3689=AXIS2_PLACEMENT_3D('',#5317,#4289,#4290);
#3690=AXIS2_PLACEMENT_3D('',#5319,#4292,#4293);
#3691=AXIS2_PLACEMENT_3D('',#5320,#4294,#4295);
#3692=AXIS2_PLACEMENT_3D('',#5333,#4302,#4303);
#3693=AXIS2_PLACEMENT_3D('',#5334,#4304,#4305);
#3694=AXIS2_PLACEMENT_3D('',#5336,#4307,#4308);
#3695=AXIS2_PLACEMENT_3D('',#5337,#4309,#4310);
#3696=AXIS2_PLACEMENT_3D('',#5343,#4316,#4317);
#3697=AXIS2_PLACEMENT_3D('',#5345,#4319,#4320);
#3698=AXIS2_PLACEMENT_3D('',#5347,#4322,#4323);
#3699=AXIS2_PLACEMENT_3D('',#5349,#4325,#4326);
#3700=AXIS2_PLACEMENT_3D('',#5351,#4328,#4329);
#3701=AXIS2_PLACEMENT_3D('',#5353,#4331,#4332);
#3702=AXIS2_PLACEMENT_3D('',#5355,#4334,#4335);
#3703=AXIS2_PLACEMENT_3D('',#5357,#4337,#4338);
#3888=DIRECTION('axis',(0.,0.,1.));
#3889=DIRECTION('refdir',(1.,0.,0.));
#3890=DIRECTION('center_axis',(0.,-0.0208291764396898,0.999783049170591));
#3891=DIRECTION('ref_axis',(1.,0.,0.));
#3892=DIRECTION('',(-1.,0.,0.));
#3893=DIRECTION('center_axis',(0.,0.0208291764396898,-0.999783049170591));
#3894=DIRECTION('ref_axis',(1.,0.,0.));
#3895=DIRECTION('center_axis',(0.,0.0208291764396898,-0.999783049170591));
#3896=DIRECTION('ref_axis',(1.,0.,0.));
#3897=DIRECTION('center_axis',(0.,0.,-1.));
#3898=DIRECTION('ref_axis',(0.,-1.,0.));
#3899=DIRECTION('',(0.,0.0208291764396898,-0.999783049170591));
#3900=DIRECTION('center_axis',(0.,0.0208291764396907,0.999783049170591));
#3901=DIRECTION('ref_axis',(0.,-0.999783049170591,0.0208291764396907));
#3902=DIRECTION('center_axis',(0.,0.0208291764396907,0.999783049170591));
#3903=DIRECTION('ref_axis',(0.,-0.999783049170591,0.0208291764396907));
#3904=DIRECTION('center_axis',(0.,0.0208291764396898,-0.999783049170591));
#3905=DIRECTION('ref_axis',(1.,0.,0.));
#3906=DIRECTION('center_axis',(0.,0.0208291764396907,-0.999783049170591));
#3907=DIRECTION('ref_axis',(1.,0.,0.));
#3908=DIRECTION('',(0.,0.0208291764396898,-0.999783049170591));
#3909=DIRECTION('center_axis',(0.,0.,1.));
#3910=DIRECTION('ref_axis',(0.,-1.,0.));
#3911=DIRECTION('center_axis',(2.44876222201709E-16,-0.0208291764396898,
-0.999783049170591));
#3912=DIRECTION('ref_axis',(1.,-7.39048179408127E-33,2.44929359829471E-16));
#3913=DIRECTION('center_axis',(0.,0.,-1.));
#3914=DIRECTION('ref_axis',(0.,-1.,0.));
#3915=DIRECTION('center_axis',(4.67925299296849E-22,-0.707104673835204,
-0.707108888531611));
#3916=DIRECTION('ref_axis',(-1.73190695094883E-16,-0.707108888531611,0.707104673835204));
#3917=DIRECTION('center_axis',(0.,0.,-1.));
#3918=DIRECTION('ref_axis',(0.,-1.,0.));
#3919=DIRECTION('',(2.44876222201709E-16,-0.0208291764396898,-0.999783049170591));
#3920=DIRECTION('center_axis',(0.,0.,1.));
#3921=DIRECTION('ref_axis',(0.,-1.,0.));
#3922=DIRECTION('center_axis',(0.,0.,-1.));
#3923=DIRECTION('ref_axis',(1.,0.,0.));
#3924=DIRECTION('',(-1.,-6.61748276614988E-22,0.));
#3925=DIRECTION('',(0.,-1.,0.));
#3926=DIRECTION('',(-1.,0.,0.));
#3927=DIRECTION('',(0.,-1.,0.));
#3928=DIRECTION('',(-1.,-6.61748276614988E-22,0.));
#3929=DIRECTION('center_axis',(0.,1.,0.));
#3930=DIRECTION('ref_axis',(1.,0.,0.));
#3931=DIRECTION('center_axis',(0.,1.,0.));
#3932=DIRECTION('ref_axis',(1.,0.,0.));
#3933=DIRECTION('',(0.,1.,0.));
#3934=DIRECTION('center_axis',(0.,1.,0.));
#3935=DIRECTION('ref_axis',(1.,0.,0.));
#3936=DIRECTION('center_axis',(0.,-1.,0.));
#3937=DIRECTION('ref_axis',(1.,0.,0.));
#3938=DIRECTION('center_axis',(0.,1.,0.));
#3939=DIRECTION('ref_axis',(1.,0.,0.));
#3940=DIRECTION('center_axis',(0.,1.,0.));
#3941=DIRECTION('ref_axis',(1.,0.,0.));
#3942=DIRECTION('',(0.,1.,0.));
#3943=DIRECTION('center_axis',(0.,1.,0.));
#3944=DIRECTION('ref_axis',(1.,0.,0.));
#3945=DIRECTION('center_axis',(0.,-1.,0.));
#3946=DIRECTION('ref_axis',(1.,0.,0.));
#3947=DIRECTION('center_axis',(-1.,0.,0.));
#3948=DIRECTION('ref_axis',(0.,0.,-1.));
#3949=DIRECTION('',(0.,0.,1.));
#3950=DIRECTION('',(-1.7319121124633E-16,-0.707108888531611,0.707104673835204));
#3951=DIRECTION('',(-1.22464679914735E-16,-1.,0.));
#3952=DIRECTION('',(1.11022302462516E-16,0.,-1.));
#3953=DIRECTION('',(0.,1.,0.));
#3954=DIRECTION('center_axis',(-1.,0.,0.));
#3955=DIRECTION('ref_axis',(0.,0.,-1.));
#3956=DIRECTION('',(0.,0.,1.));
#3957=DIRECTION('',(0.,-1.,0.));
#3958=DIRECTION('',(1.11022302462516E-16,0.,-1.));
#3959=DIRECTION('',(1.22464679914735E-16,1.,0.));
#3960=DIRECTION('',(5.16151446404829E-22,0.707108888531611,0.707104673835204));
#3961=DIRECTION('',(0.,-1.,0.));
#3962=DIRECTION('center_axis',(0.,0.,-1.));
#3963=DIRECTION('ref_axis',(1.,0.,0.));
#3964=DIRECTION('',(1.,0.,-2.64892773006431E-15));
#3965=DIRECTION('',(0.,-1.,0.));
#3966=DIRECTION('',(0.,-1.,0.));
#3967=DIRECTION('',(1.,0.,0.));
#3968=DIRECTION('center_axis',(0.,1.,0.));
#3969=DIRECTION('ref_axis',(1.,0.,0.));
#3970=DIRECTION('center_axis',(0.,-1.,0.));
#3971=DIRECTION('ref_axis',(1.,0.,0.));
#3972=DIRECTION('center_axis',(0.,-1.,0.));
#3973=DIRECTION('ref_axis',(1.,0.,0.));
#3974=DIRECTION('',(0.,-1.,0.));
#3975=DIRECTION('center_axis',(0.,1.,0.));
#3976=DIRECTION('ref_axis',(1.,0.,0.));
#3977=DIRECTION('center_axis',(2.63841010085458E-15,0.,1.));
#3978=DIRECTION('ref_axis',(-1.,0.,2.63841010085458E-15));
#3979=DIRECTION('',(1.,0.,-2.63841010085458E-15));
#3980=DIRECTION('',(0.,-1.,0.));
#3981=DIRECTION('',(1.,0.,7.37272213361077E-17));
#3982=DIRECTION('',(0.,-1.,0.));
#3983=DIRECTION('',(-1.,0.,-7.37272213361077E-17));
#3984=DIRECTION('center_axis',(1.,0.,0.));
#3985=DIRECTION('ref_axis',(0.,0.,1.));
#3986=DIRECTION('',(0.,0.,-1.));
#3987=DIRECTION('',(0.,-1.,0.));
#3988=DIRECTION('',(0.,0.,1.));
#3989=DIRECTION('',(0.,-1.,0.));
#3990=DIRECTION('center_axis',(0.,-1.,0.));
#3991=DIRECTION('ref_axis',(-1.77635683940025E-15,0.,-1.));
#3992=DIRECTION('center_axis',(0.,-1.,0.));
#3993=DIRECTION('ref_axis',(-1.77635683940025E-15,0.,-1.));
#3994=DIRECTION('center_axis',(0.,1.,0.));
#3995=DIRECTION('ref_axis',(-1.77635683940025E-15,0.,-1.));
#3996=DIRECTION('center_axis',(0.,-1.,0.));
#3997=DIRECTION('ref_axis',(-1.99840144432528E-15,0.,-1.));
#3998=DIRECTION('center_axis',(0.,1.,0.));
#3999=DIRECTION('ref_axis',(-1.99840144432528E-15,0.,-1.));
#4000=DIRECTION('center_axis',(0.,-1.,0.));
#4001=DIRECTION('ref_axis',(-1.99840144432528E-15,0.,-1.));
#4002=DIRECTION('',(0.,-1.,0.));
#4003=DIRECTION('center_axis',(-1.,0.,0.));
#4004=DIRECTION('ref_axis',(0.,0.,-1.));
#4005=DIRECTION('',(0.,0.,-1.));
#4006=DIRECTION('',(0.,0.,-1.));
#4007=DIRECTION('',(0.,-1.,0.));
#4008=DIRECTION('center_axis',(-1.11022302462516E-16,1.35963107344689E-32,
1.));
#4009=DIRECTION('ref_axis',(1.22464679914735E-16,1.,1.64214663788065E-47));
#4010=DIRECTION('',(-1.,0.,-1.11022302462516E-16));
#4011=DIRECTION('',(-1.22464679914735E-16,-1.,0.));
#4012=DIRECTION('',(-1.,1.22464679914735E-16,-1.11022302462516E-16));
#4013=DIRECTION('center_axis',(-1.65100204443931E-16,-0.707104673835204,
0.707108888531611));
#4014=DIRECTION('ref_axis',(5.16151446398137E-22,0.707108888531611,0.707104673835204));
#4015=DIRECTION('',(-5.16151446404829E-22,-0.707108888531611,-0.707104673835204));
#4016=DIRECTION('',(1.,-2.33487644125528E-16,0.));
#4017=DIRECTION('center_axis',(4.67925299296849E-22,-0.707104673835204,
-0.707108888531611));
#4018=DIRECTION('ref_axis',(-1.7319121124633E-16,-0.707108888531611,0.707104673835204));
#4019=DIRECTION('',(1.7319121124633E-16,0.707108888531611,-0.707104673835204));
#4020=DIRECTION('',(-1.,1.11022302462516E-16,-1.11022302462516E-16));
#4021=DIRECTION('center_axis',(1.11022302462516E-16,-1.35963107344689E-32,
-1.));
#4022=DIRECTION('ref_axis',(-1.22464679914735E-16,-1.,-1.64214663788065E-47));
#4023=DIRECTION('',(1.22464679914735E-16,1.,0.));
#4024=DIRECTION('',(1.,0.,1.11022302462516E-16));
#4025=DIRECTION('center_axis',(0.,1.,0.));
#4026=DIRECTION('ref_axis',(1.,0.,0.));
#4027=DIRECTION('',(1.,0.,0.));
#4028=DIRECTION('',(0.,0.,-1.));
#4029=DIRECTION('',(1.,0.,-2.64892773006431E-15));
#4030=DIRECTION('center_axis',(0.,-1.,0.));
#4031=DIRECTION('ref_axis',(0.707106824182887,0.,0.707106738190206));
#4032=DIRECTION('',(-1.,0.,-7.37272213361077E-17));
#4033=DIRECTION('',(0.,0.,-1.));
#4034=DIRECTION('center_axis',(0.,-1.,0.));
#4035=DIRECTION('ref_axis',(-0.192330993613605,0.,0.981330112090526));
#4036=DIRECTION('center_axis',(0.,-1.,0.));
#4037=DIRECTION('ref_axis',(-0.192330993613605,0.,0.981330112090526));
#4038=DIRECTION('',(0.,-1.,0.));
#4039=DIRECTION('center_axis',(0.,1.,0.));
#4040=DIRECTION('ref_axis',(-0.192330993613605,0.,0.981330112090526));
#4041=DIRECTION('center_axis',(1.,0.,0.));
#4042=DIRECTION('ref_axis',(0.,0.,1.));
#4043=DIRECTION('',(0.,-1.,0.));
#4044=DIRECTION('',(0.,0.,1.));
#4045=DIRECTION('center_axis',(0.,0.,1.));
#4046=DIRECTION('ref_axis',(-1.,0.,0.));
#4047=DIRECTION('',(0.,-1.,0.));
#4048=DIRECTION('center_axis',(1.,0.,0.));
#4049=DIRECTION('ref_axis',(0.,0.,1.));
#4050=DIRECTION('',(-1.11022302462516E-16,0.,1.));
#4051=DIRECTION('',(0.,1.,0.));
#4052=DIRECTION('center_axis',(2.63841010085458E-15,0.,1.));
#4053=DIRECTION('ref_axis',(-1.,0.,2.63841010085458E-15));
#4054=DIRECTION('',(0.,-1.,0.));
#4055=DIRECTION('',(1.,0.,7.37272213361077E-17));
#4056=DIRECTION('',(0.,-1.,0.));
#4057=DIRECTION('',(1.,0.,-2.63841010085458E-15));
#4058=DIRECTION('center_axis',(0.,-1.,0.));
#4059=DIRECTION('ref_axis',(0.999999975140088,0.,0.000222979425697669));
#4060=DIRECTION('center_axis',(0.,-1.,0.));
#4061=DIRECTION('ref_axis',(0.999999975140088,0.,0.000222979425697669));
#4062=DIRECTION('center_axis',(0.,1.,0.));
#4063=DIRECTION('ref_axis',(0.999999975140088,0.,0.000222979425697669));
#4064=DIRECTION('',(0.,-1.,0.));
#4065=DIRECTION('center_axis',(-0.999999975140088,0.,-0.000222979425718608));
#4066=DIRECTION('ref_axis',(0.000222979425718608,0.,-0.999999975140088));
#4067=DIRECTION('',(-0.000222979425718608,0.,0.999999975140088));
#4068=DIRECTION('',(0.000222979425718608,0.,-0.999999975140088));
#4069=DIRECTION('',(0.,-1.,0.));
#4070=DIRECTION('center_axis',(0.,-1.,0.));
#4071=DIRECTION('ref_axis',(-0.149925588670012,0.,0.988697283227758));
#4072=DIRECTION('center_axis',(0.,-1.,0.));
#4073=DIRECTION('ref_axis',(-0.149925588670012,0.,0.988697283227758));
#4074=DIRECTION('center_axis',(0.,1.,0.));
#4075=DIRECTION('ref_axis',(-0.149925588670012,0.,0.988697283227758));
#4076=DIRECTION('center_axis',(0.602735860859126,0.,0.797940776019379));
#4077=DIRECTION('ref_axis',(-0.797940776019379,0.,0.602735860859126));
#4078=DIRECTION('',(0.797940776019378,0.,-0.602735860859126));
#4079=DIRECTION('',(-0.797940776019378,0.,0.602735860859126));
#4080=DIRECTION('',(0.,-1.,0.));
#4081=DIRECTION('center_axis',(0.,-1.,0.));
#4082=DIRECTION('ref_axis',(0.619814087082361,0.,0.784748684264115));
#4083=DIRECTION('center_axis',(0.,1.,0.));
#4084=DIRECTION('ref_axis',(0.619814087082361,0.,0.784748684264115));
#4085=DIRECTION('center_axis',(0.,-1.,0.));
#4086=DIRECTION('ref_axis',(0.619814087082361,0.,0.784748684264115));
#4087=DIRECTION('',(0.,-1.,0.));
#4088=DIRECTION('center_axis',(1.,0.,0.));
#4089=DIRECTION('ref_axis',(0.,0.,1.));
#4090=DIRECTION('',(0.,0.,1.));
#4091=DIRECTION('',(0.,0.,1.));
#4092=DIRECTION('',(0.,-1.,0.));
#4093=DIRECTION('center_axis',(0.,-1.,0.));
#4094=DIRECTION('ref_axis',(0.382683511888619,0.,-0.923879499571558));
#4095=DIRECTION('center_axis',(0.,1.,0.));
#4096=DIRECTION('ref_axis',(0.70710688994201,0.,0.707106672431068));
#4097=DIRECTION('center_axis',(0.,1.,0.));
#4098=DIRECTION('ref_axis',(0.70710688994201,0.,0.707106672431068));
#4099=DIRECTION('',(0.,1.,0.));
#4100=DIRECTION('center_axis',(0.,0.,-1.));
#4101=DIRECTION('ref_axis',(1.,0.,0.));
#4102=DIRECTION('',(1.,0.,0.));
#4103=DIRECTION('',(0.,-1.,0.));
#4104=DIRECTION('',(0.,-1.,0.));
#4105=DIRECTION('center_axis',(0.,-1.,0.));
#4106=DIRECTION('ref_axis',(0.707106824182887,0.,0.707106738190205));
#4107=DIRECTION('center_axis',(0.,1.,0.));
#4108=DIRECTION('ref_axis',(0.707106824182887,0.,0.707106738190205));
#4109=DIRECTION('',(0.,-1.,0.));
#4110=DIRECTION('center_axis',(0.,-1.,0.));
#4111=DIRECTION('ref_axis',(0.707106824182887,0.,0.707106738190205));
#4112=DIRECTION('center_axis',(0.,-1.,0.));
#4113=DIRECTION('ref_axis',(-0.70710688994201,0.,-0.707106672431068));
#4114=DIRECTION('center_axis',(0.,1.,0.));
#4115=DIRECTION('ref_axis',(-0.70710688994201,0.,-0.707106672431068));
#4116=DIRECTION('',(0.,-1.,0.));
#4117=DIRECTION('center_axis',(0.,-1.,0.));
#4118=DIRECTION('ref_axis',(-0.70710688994201,0.,-0.707106672431068));
#4119=DIRECTION('center_axis',(0.,-1.,0.));
#4120=DIRECTION('ref_axis',(-0.70710688994201,0.,-0.707106672431068));
#4121=DIRECTION('',(0.,-1.,0.));
#4122=DIRECTION('center_axis',(0.707106955701123,0.,0.707106606671929));
#4123=DIRECTION('ref_axis',(-0.707106606671929,0.,0.707106955701123));
#4124=DIRECTION('',(0.707106606671929,0.,-0.707106955701123));
#4125=DIRECTION('',(0.,-1.,0.));
#4126=DIRECTION('',(-0.707106606671929,0.,0.707106955701123));
#4127=DIRECTION('center_axis',(0.,-1.,0.));
#4128=DIRECTION('ref_axis',(-0.382683511888619,0.,0.923879499571558));
#4129=DIRECTION('center_axis',(0.,1.,0.));
#4130=DIRECTION('ref_axis',(-0.70710688994201,0.,-0.707106672431068));
#4131=DIRECTION('',(0.,-1.,0.));
#4132=DIRECTION('center_axis',(0.,1.,0.));
#4133=DIRECTION('ref_axis',(-0.70710688994201,0.,-0.707106672431068));
#4134=DIRECTION('center_axis',(-1.,0.,0.));
#4135=DIRECTION('ref_axis',(0.,0.,-1.));
#4136=DIRECTION('',(0.,0.,-1.));
#4137=DIRECTION('',(0.,-1.,0.));
#4138=DIRECTION('',(0.,0.,-1.));
#4139=DIRECTION('center_axis',(0.,-1.,0.));
#4140=DIRECTION('ref_axis',(-0.619814087082361,0.,-0.784748684264115));
#4141=DIRECTION('center_axis',(0.,1.,0.));
#4142=DIRECTION('ref_axis',(-0.619814087082361,0.,-0.784748684264115));
#4143=DIRECTION('',(0.,-1.,0.));
#4144=DIRECTION('center_axis',(0.,-1.,0.));
#4145=DIRECTION('ref_axis',(-0.619814087082361,0.,-0.784748684264115));
#4146=DIRECTION('center_axis',(0.999999975140088,0.,0.000222979425718608));
#4147=DIRECTION('ref_axis',(-0.000222979425718608,0.,0.999999975140088));
#4148=DIRECTION('',(0.000222979425718608,0.,-0.999999975140088));
#4149=DIRECTION('',(0.,-1.,0.));
#4150=DIRECTION('',(-0.000222979425718608,0.,0.999999975140088));
#4151=DIRECTION('',(0.,-1.,0.));
#4152=DIRECTION('center_axis',(0.,-1.,0.));
#4153=DIRECTION('ref_axis',(-0.999999975140088,0.,-0.000222979425691007));
#4154=DIRECTION('center_axis',(0.,-1.,0.));
#4155=DIRECTION('ref_axis',(-0.999999975140088,0.,-0.000222979425691007));
#4156=DIRECTION('',(0.,-1.,0.));
#4157=DIRECTION('center_axis',(0.,1.,0.));
#4158=DIRECTION('ref_axis',(-0.999999975140088,0.,-0.000222979425691007));
#4159=DIRECTION('center_axis',(0.,-1.,0.));
#4160=DIRECTION('ref_axis',(-0.707106824182888,0.,-0.707106738190205));
#4161=DIRECTION('',(0.,-1.,0.));
#4162=DIRECTION('center_axis',(0.,-1.,0.));
#4163=DIRECTION('ref_axis',(-0.707106824182888,0.,-0.707106738190205));
#4164=DIRECTION('',(0.,-1.,0.));
#4165=DIRECTION('center_axis',(-1.,0.,0.));
#4166=DIRECTION('ref_axis',(0.,0.,1.));
#4167=DIRECTION('',(0.,0.,1.));
#4168=DIRECTION('',(0.,-1.,0.));
#4169=DIRECTION('',(0.,0.,1.));
#4170=DIRECTION('',(0.,1.,0.));
#4171=DIRECTION('center_axis',(-1.,0.,0.));
#4172=DIRECTION('ref_axis',(0.,0.,1.));
#4173=DIRECTION('',(0.,0.,1.));
#4174=DIRECTION('',(0.,1.,0.));
#4175=DIRECTION('',(0.,0.,1.));
#4176=DIRECTION('',(0.,1.,0.));
#4177=DIRECTION('center_axis',(-1.,0.,0.));
#4178=DIRECTION('ref_axis',(0.,0.,1.));
#4179=DIRECTION('',(0.,0.,1.));
#4180=DIRECTION('',(0.,0.999783049170591,0.0208291764396907));
#4181=DIRECTION('',(0.,0.,1.));
#4182=DIRECTION('',(0.,-1.,0.));
#4183=DIRECTION('',(0.,-0.707108888531611,-0.707104673835204));
#4184=DIRECTION('',(0.,-0.707108888531611,0.707104673835204));
#4185=DIRECTION('center_axis',(-1.,0.,0.));
#4186=DIRECTION('ref_axis',(0.,0.,1.));
#4187=DIRECTION('',(0.,0.,1.));
#4188=DIRECTION('',(0.,0.707108888531611,0.707104673835204));
#4189=DIRECTION('',(0.,0.707108888531611,-0.707104673835204));
#4190=DIRECTION('',(0.,1.,0.));
#4191=DIRECTION('',(0.,0.,1.));
#4192=DIRECTION('',(0.,-0.999783049170591,0.0208291764396907));
#4193=DIRECTION('center_axis',(-0.707106889942011,0.,-0.707106672431068));
#4194=DIRECTION('ref_axis',(0.707106672431068,0.,-0.707106889942011));
#4195=DIRECTION('',(0.707106672431068,0.,-0.70710688994201));
#4196=DIRECTION('',(0.707106672431068,0.,-0.70710688994201));
#4197=DIRECTION('center_axis',(0.,-1.,0.));
#4198=DIRECTION('ref_axis',(0.192330993613606,0.,-0.981330112090525));
#4199=DIRECTION('center_axis',(0.,1.,0.));
#4200=DIRECTION('ref_axis',(0.192330993613606,0.,-0.981330112090525));
#4201=DIRECTION('',(0.,-1.,0.));
#4202=DIRECTION('center_axis',(0.,-1.,0.));
#4203=DIRECTION('ref_axis',(0.192330993613606,0.,-0.981330112090525));
#4204=DIRECTION('center_axis',(1.,0.,0.));
#4205=DIRECTION('ref_axis',(0.,0.,1.));
#4206=DIRECTION('',(0.,0.,-1.));
#4207=DIRECTION('',(0.,-1.,0.));
#4208=DIRECTION('',(0.,0.,1.));
#4209=DIRECTION('center_axis',(0.,-1.,0.));
#4210=DIRECTION('ref_axis',(0.,0.,1.));
#4211=DIRECTION('center_axis',(0.,1.,0.));
#4212=DIRECTION('ref_axis',(0.,0.,1.));
#4213=DIRECTION('',(0.,-1.,0.));
#4214=DIRECTION('center_axis',(0.,-1.,0.));
#4215=DIRECTION('ref_axis',(0.,0.,1.));
#4216=DIRECTION('',(0.,-1.,0.));
#4217=DIRECTION('center_axis',(0.,0.,1.));
#4218=DIRECTION('ref_axis',(-1.,0.,0.));
#4219=DIRECTION('',(1.,0.,0.));
#4220=DIRECTION('',(1.,0.,0.));
#4221=DIRECTION('',(0.,-1.,0.));
#4222=DIRECTION('',(-1.,0.,2.56034438634048E-15));
#4223=DIRECTION('',(-1.,0.,0.));
#4224=DIRECTION('',(-1.,0.,2.56034438634048E-15));
#4225=DIRECTION('',(1.,0.,0.));
#4226=DIRECTION('center_axis',(0.,-1.,0.));
#4227=DIRECTION('ref_axis',(0.,0.,1.));
#4228=DIRECTION('center_axis',(0.,-1.,0.));
#4229=DIRECTION('ref_axis',(0.,0.,1.));
#4230=DIRECTION('',(0.,-1.,0.));
#4231=DIRECTION('center_axis',(0.,1.,0.));
#4232=DIRECTION('ref_axis',(0.,0.,1.));
#4233=DIRECTION('',(0.,-1.,0.));
#4234=DIRECTION('center_axis',(-1.,0.,0.));
#4235=DIRECTION('ref_axis',(0.,0.,-1.));
#4236=DIRECTION('',(0.,0.,1.));
#4237=DIRECTION('',(0.,-1.,0.));
#4238=DIRECTION('',(0.,0.,-1.));
#4239=DIRECTION('center_axis',(0.,1.,0.));
#4240=DIRECTION('ref_axis',(1.,0.,0.));
#4241=DIRECTION('',(-1.,0.,2.63527591935953E-15));
#4242=DIRECTION('center_axis',(0.,1.,0.));
#4243=DIRECTION('ref_axis',(0.149925588670012,0.,-0.988697283227758));
#4244=DIRECTION('',(-1.,0.,2.63527591935953E-15));
#4245=DIRECTION('center_axis',(0.,-1.,0.));
#4246=DIRECTION('ref_axis',(1.,0.,0.));
#4247=DIRECTION('center_axis',(0.,-1.,0.));
#4248=DIRECTION('ref_axis',(1.,0.,0.));
#4249=DIRECTION('',(0.,-1.,0.));
#4250=DIRECTION('center_axis',(0.,1.,0.));
#4251=DIRECTION('ref_axis',(1.,0.,0.));
#4252=DIRECTION('center_axis',(0.,1.,0.));
#4253=DIRECTION('ref_axis',(1.,0.,0.));
#4254=DIRECTION('center_axis',(1.,0.,0.));
#4255=DIRECTION('ref_axis',(0.,0.,-1.));
#4256=DIRECTION('',(0.,0.,-1.));
#4257=DIRECTION('',(0.,1.,0.));
#4258=DIRECTION('',(0.,0.,-1.));
#4259=DIRECTION('',(0.,1.,0.));
#4260=DIRECTION('center_axis',(0.,1.,0.));
#4261=DIRECTION('ref_axis',(0.,0.,1.));
#4262=DIRECTION('',(-1.,0.,0.));
#4263=DIRECTION('',(0.,0.,-1.));
#4264=DIRECTION('',(0.,0.,-1.));
#4265=DIRECTION('',(-1.,0.,0.));
#4266=DIRECTION('center_axis',(1.,0.,0.));
#4267=DIRECTION('ref_axis',(0.,0.,-1.));
#4268=DIRECTION('',(0.,0.,-1.));
#4269=DIRECTION('',(0.,1.,0.));
#4270=DIRECTION('center_axis',(0.,0.,-1.));
#4271=DIRECTION('ref_axis',(-1.,0.,0.));
#4272=DIRECTION('',(-1.,0.,0.));
#4273=DIRECTION('center_axis',(0.,-1.,0.));
#4274=DIRECTION('ref_axis',(0.,0.,1.));
#4275=DIRECTION('',(1.,0.,0.));
#4276=DIRECTION('',(0.,0.,-1.));
#4277=DIRECTION('',(-1.,0.,0.));
#4278=DIRECTION('center_axis',(0.,-0.0208291764396907,0.999783049170591));
#4279=DIRECTION('ref_axis',(0.,0.999783049170591,0.0208291764396907));
#4280=DIRECTION('',(0.,-0.999783049170591,-0.0208291764396907));
#4281=DIRECTION('center_axis',(0.,0.,-1.));
#4282=DIRECTION('ref_axis',(0.,-1.,0.));
#4283=DIRECTION('',(0.,1.,0.));
#4284=DIRECTION('',(-1.,0.,0.));
#4285=DIRECTION('center_axis',(0.,0.707104673835204,-0.707108888531611));
#4286=DIRECTION('ref_axis',(0.,-0.707108888531611,-0.707104673835204));
#4287=DIRECTION('',(0.,0.707108888531611,0.707104673835204));
#4288=DIRECTION('',(-1.,0.,0.));
#4289=DIRECTION('center_axis',(0.,-0.707104673835204,-0.707108888531611));
#4290=DIRECTION('ref_axis',(0.,-0.707108888531611,0.707104673835204));
#4291=DIRECTION('',(0.,0.707108888531611,-0.707104673835204));
#4292=DIRECTION('center_axis',(1.,0.,0.));
#4293=DIRECTION('ref_axis',(0.,0.,-1.));
#4294=DIRECTION('center_axis',(1.,0.,0.));
#4295=DIRECTION('ref_axis',(0.,0.,-1.));
#4296=DIRECTION('',(0.,0.,-1.));
#4297=DIRECTION('',(0.,0.999783049170591,-0.0208291764396907));
#4298=DIRECTION('',(0.,0.,-1.));
#4299=DIRECTION('',(0.,-1.,0.));
#4300=DIRECTION('',(0.,-0.707108888531611,0.707104673835204));
#4301=DIRECTION('',(0.,-0.707108888531611,-0.707104673835204));
#4302=DIRECTION('center_axis',(0.,1.,0.));
#4303=DIRECTION('ref_axis',(1.,0.,0.));
#4304=DIRECTION('center_axis',(0.,-1.,0.));
#4305=DIRECTION('ref_axis',(0.149925588670012,0.,-0.988697283227758));
#4306=DIRECTION('',(-1.,0.,2.72352010410795E-15));
#4307=DIRECTION('center_axis',(0.,-1.,0.));
#4308=DIRECTION('ref_axis',(0.149925588670012,0.,-0.988697283227758));
#4309=DIRECTION('center_axis',(-2.72352010410795E-15,0.,-1.));
#4310=DIRECTION('ref_axis',(1.,0.,-2.72352010410795E-15));
#4311=DIRECTION('',(1.,0.,-2.63527591935953E-15));
#4312=DIRECTION('',(-1.,0.,2.72352010410795E-15));
#4313=DIRECTION('',(-1.,0.,2.72352010410795E-15));
#4314=DIRECTION('',(-1.,0.,2.72352010410795E-15));
#4315=DIRECTION('',(1.,0.,-2.63527591935953E-15));
#4316=DIRECTION('center_axis',(0.,-0.0208291764396907,-0.999783049170591));
#4317=DIRECTION('ref_axis',(0.,-0.999783049170591,0.0208291764396907));
#4318=DIRECTION('',(1.,0.,0.));
#4319=DIRECTION('center_axis',(0.,-1.,0.));
#4320=DIRECTION('ref_axis',(0.,0.,1.));
#4321=DIRECTION('',(-1.,0.,0.));
#4322=DIRECTION('center_axis',(0.,-0.707104673835204,0.707108888531611));
#4323=DIRECTION('ref_axis',(0.,0.707108888531611,0.707104673835204));
#4324=DIRECTION('',(-1.,0.,0.));
#4325=DIRECTION('center_axis',(0.,0.707104673835204,0.707108888531611));
#4326=DIRECTION('ref_axis',(0.,0.707108888531611,-0.707104673835204));
#4327=DIRECTION('',(-1.,0.,0.));
#4328=DIRECTION('center_axis',(0.,0.,1.));
#4329=DIRECTION('ref_axis',(0.,1.,0.));
#4330=DIRECTION('',(1.,0.,0.));
#4331=DIRECTION('center_axis',(0.,1.,0.));
#4332=DIRECTION('ref_axis',(0.,0.,1.));
#4333=DIRECTION('',(1.,0.,0.));
#4334=DIRECTION('center_axis',(0.,0.,1.));
#4335=DIRECTION('ref_axis',(1.,0.,0.));
#4336=DIRECTION('',(1.,0.,0.));
#4337=DIRECTION('center_axis',(0.,1.,0.));
#4338=DIRECTION('ref_axis',(1.,0.,0.));
#4890=CARTESIAN_POINT('',(0.,0.,0.));
#4891=CARTESIAN_POINT('Origin',(55.4902124404907,-11.9018738839031,101.14418999359));
#4892=CARTESIAN_POINT('',(56.823388803725,-10.4113449571108,101.175243220618));
#4893=CARTESIAN_POINT('',(54.1570360772564,-10.4113449571108,101.175243220618));
#4894=CARTESIAN_POINT('',(55.4902124404907,-10.4113449571108,101.175243220618));
#4895=CARTESIAN_POINT('Origin',(55.4902124404907,-11.9018738839031,101.14418999359));
#4896=CARTESIAN_POINT('Origin',(55.4902124404907,-12.0000001341105,105.854167938232));
#4897=CARTESIAN_POINT('',(53.4902124404907,-11.9197037286391,102.000007629395));
#4898=CARTESIAN_POINT('Origin',(55.4902124404907,-11.9197037286391,102.000007629395));
#4899=CARTESIAN_POINT('',(53.4902124404907,-11.9031683527619,101.206323416217));
#4900=CARTESIAN_POINT('',(53.4902124404907,-12.0000001341105,105.854167938232));
#4901=CARTESIAN_POINT('Origin',(55.4902124404907,-11.9031683527619,101.206323416217));
#4902=CARTESIAN_POINT('Origin',(55.4902124404907,-11.9031683527619,101.206323416217));
#4903=CARTESIAN_POINT('Origin',(55.4902124404907,-12.0000001341105,105.854167938232));
#4904=CARTESIAN_POINT('',(53.4902124404907,-11.998698570337,105.791693965635));
#4905=CARTESIAN_POINT('Origin',(55.4902124404907,-11.998698570337,105.791693965635));
#4906=CARTESIAN_POINT('',(53.4902124404907,-11.9822046586727,105.));
#4907=CARTESIAN_POINT('',(53.4902124404907,-12.0000001341105,105.854167938232));
#4908=CARTESIAN_POINT('Origin',(55.4902124404907,-11.9822046586727,105.));
#4909=CARTESIAN_POINT('Origin',(55.4902124404907,-4.00000013411045,0.145828066207017));
#4910=CARTESIAN_POINT('',(55.5312016298222,-1.92132882178138,3.92132133245468));
#4911=CARTESIAN_POINT('',(53.4902124404907,-3.92134265391535,3.92132133245468));
#4912=CARTESIAN_POINT('Origin',(55.4902124404907,-3.92134265391535,3.92132133245468));
#4913=CARTESIAN_POINT('',(55.4492232511593,-1.92132882178138,3.92132133245468));
#4914=CARTESIAN_POINT('Origin',(55.4902124404907,-3.88052558675829,5.88050641971165));
#4915=CARTESIAN_POINT('Origin',(55.4902124404907,-3.92134265391535,3.92132133245468));
#4916=CARTESIAN_POINT('',(53.4902124404907,-3.97803783517153,1.20000004768372));
#4917=CARTESIAN_POINT('',(53.4902124404907,-4.00000013411045,0.145828066207016));
#4918=CARTESIAN_POINT('Origin',(55.4902124404907,-3.97803783517153,1.20000004768372));
#4919=CARTESIAN_POINT('Origin',(50.4902124404907,0.,3.92132133245468));
#4920=CARTESIAN_POINT('',(50.4902111949968,-1.92132882178138,3.92132133245468));
#4921=CARTESIAN_POINT('',(52.9902111948072,-1.92132882178138,3.92132133245468));
#4922=CARTESIAN_POINT('',(50.4902124404907,-8.,3.92132133245468));
#4923=CARTESIAN_POINT('',(50.4902124404907,0.,3.92132133245468));
#4924=CARTESIAN_POINT('',(60.4902124404907,-8.,3.92132133245468));
#4925=CARTESIAN_POINT('',(51.5279682097109,-8.,3.92132133245468));
#4926=CARTESIAN_POINT('',(60.4902111949968,-1.92132882178138,3.92132133245468));
#4927=CARTESIAN_POINT('',(60.4902124404907,0.,3.92132133245468));
#4928=CARTESIAN_POINT('',(52.9902111948072,-1.92132882178138,3.92132133245468));
#4929=CARTESIAN_POINT('Origin',(10.0000045479708,-8.,103.499999046326));
#4930=CARTESIAN_POINT('',(8.50000441279955,-8.,103.499999046326));
#4931=CARTESIAN_POINT('Origin',(10.0000045479708,-8.,103.499999046326));
#4932=CARTESIAN_POINT('',(8.50000441279955,-2.8,103.499999046326));
#4933=CARTESIAN_POINT('',(8.50000441279957,-8.,103.499999046326));
#4934=CARTESIAN_POINT('Origin',(10.0000045479708,-2.8,103.499999046326));
#4935=CARTESIAN_POINT('Origin',(10.0000045479708,-2.8,103.499999046326));
#4936=CARTESIAN_POINT('Origin',(100.979996788778,-8.,2.49999516053467));
#4937=CARTESIAN_POINT('',(99.4799971640107,-8.,2.49999516053467));
#4938=CARTESIAN_POINT('Origin',(100.979996788778,-8.,2.49999516053467));
#4939=CARTESIAN_POINT('',(99.4799971640107,-2.8,2.49999516053467));
#4940=CARTESIAN_POINT('',(99.4799971640111,-8.,2.49999516053467));
#4941=CARTESIAN_POINT('Origin',(100.979996788778,-2.8,2.49999516053467));
#4942=CARTESIAN_POINT('Origin',(100.979996788778,-2.8,2.49999516053467));
#4943=CARTESIAN_POINT('Origin',(50.4902124404907,0.,4.99999999999986));
#4944=CARTESIAN_POINT('',(50.4902124404907,-8.,4.99999999999986));
#4945=CARTESIAN_POINT('',(50.4902124404907,-8.,3.74999999999986));
#4946=CARTESIAN_POINT('',(50.4902099495032,-1.00000000000001,2.99999800221971));
#4947=CARTESIAN_POINT('',(50.4902099491237,-1.00000000000001,2.99999800221971));
#4948=CARTESIAN_POINT('',(50.4902099495032,0.,2.99999800221971));
#4949=CARTESIAN_POINT('',(50.4902099491237,-1.00000000000001,2.99999800221971));
#4950=CARTESIAN_POINT('',(50.4902111949971,0.,4.99999999999986));
#4951=CARTESIAN_POINT('',(50.4902099491237,0.,28.230330787343));
#4952=CARTESIAN_POINT('',(50.4902124404907,0.,4.99999999999986));
#4953=CARTESIAN_POINT('Origin',(50.4902124404907,0.,1.20000004768372));
#4954=CARTESIAN_POINT('',(50.4902124404907,-8.,-1.59733337667944E-13));
#4955=CARTESIAN_POINT('',(50.4902124404907,-8.,1.20000004768372));
#4956=CARTESIAN_POINT('',(50.4902124404907,-8.,1.85000002384179));
#4957=CARTESIAN_POINT('',(50.4902111949971,0.,0.));
#4958=CARTESIAN_POINT('',(50.4902124404907,0.,0.));
#4959=CARTESIAN_POINT('',(50.4902099495032,0.,1.99999418752244));
#4960=CARTESIAN_POINT('',(50.4902099491237,0.,27.2999995124759));
#4961=CARTESIAN_POINT('',(50.4902099495032,-1.00000000000001,1.99999418752245));
#4962=CARTESIAN_POINT('',(50.4902099491237,1.73686967253925,1.99999418752245));
#4963=CARTESIAN_POINT('',(50.4902111949968,-1.79999890820268,1.20000004768372));
#4964=CARTESIAN_POINT('',(50.4902099491237,-2.00000023841859,0.999999909568344));
#4965=CARTESIAN_POINT('',(50.4902124404907,0.,1.20000004768372));
#4966=CARTESIAN_POINT('Origin',(5.0000011920929,0.,0.));
#4967=CARTESIAN_POINT('',(5.,-8.,-1.27675647831893E-14));
#4968=CARTESIAN_POINT('',(5.,-8.,-1.27675647831893E-14));
#4969=CARTESIAN_POINT('',(5.00000059604645,-7.,-6.38378239159465E-15));
#4970=CARTESIAN_POINT('',(5.,0.,-1.27675647831893E-14));
#4971=CARTESIAN_POINT('',(5.0000011920929,0.,0.));
#4972=CARTESIAN_POINT('',(5.0000011920929,0.,0.));
#4973=CARTESIAN_POINT('',(0.,0.,0.));
#4974=CARTESIAN_POINT('Origin',(10.0000020566037,-2.8,2.50000086324266));
#4975=CARTESIAN_POINT('',(8.25000236106051,-2.8,2.50000086324266));
#4976=CARTESIAN_POINT('Origin',(10.0000020566037,-2.8,2.50000086324266));
#4977=CARTESIAN_POINT('Origin',(10.0000020566037,0.,2.50000086324266));
#4978=CARTESIAN_POINT('',(8.25000236106051,-8.,2.50000086324266));
#4979=CARTESIAN_POINT('',(8.25000236106046,0.,2.50000086324266));
#4980=CARTESIAN_POINT('Origin',(10.0000020566037,-8.,2.50000086324266));
#4981=CARTESIAN_POINT('Origin',(75.2228282332459,0.,4.9999999999998));
#4982=CARTESIAN_POINT('',(9.99999999999999,0.,4.99999999999997));
#4983=CARTESIAN_POINT('',(9.99999999999999,0.,4.99999999999997));
#4984=CARTESIAN_POINT('',(9.99999999999999,-7.,4.99999999999997));
#4985=CARTESIAN_POINT('',(9.99999999999999,0.,4.99999999999997));
#4986=CARTESIAN_POINT('',(5.55111512312579E-15,-7.,5.00000039726821));
#4987=CARTESIAN_POINT('',(79.9288641879263,-7.,5.00000000000001));
#4988=CARTESIAN_POINT('',(1.33226762955019E-14,-8.,5.));
#4989=CARTESIAN_POINT('',(1.33226762955019E-14,0.,5.));
#4990=CARTESIAN_POINT('',(1.33226762955019E-14,-8.,5.));
#4991=CARTESIAN_POINT('Origin',(5.00000000000001,0.,9.99999999999997));
#4992=CARTESIAN_POINT('',(5.00000000000001,0.,40.7547938331316));
#4993=CARTESIAN_POINT('',(5.00000000000001,0.,9.99999999999997));
#4994=CARTESIAN_POINT('',(5.00000000000001,0.,9.99999999999997));
#4995=CARTESIAN_POINT('',(5.00000000000001,-7.,40.7547938331316));
#4996=CARTESIAN_POINT('',(5.00000000000001,0.,40.7547938331316));
#4997=CARTESIAN_POINT('',(5.00000000000001,-7.,9.99999999999997));
#4998=CARTESIAN_POINT('',(5.00000000000001,-7.,9.99999999999997));
#4999=CARTESIAN_POINT('',(5.00000000000001,0.,9.99999999999997));
#5000=CARTESIAN_POINT('Origin',(10.,0.,9.99999999999996));
#5001=CARTESIAN_POINT('Origin',(10.,0.,9.99999999999996));
#5002=CARTESIAN_POINT('Origin',(10.,-7.,9.99999999999996));
#5003=CARTESIAN_POINT('Origin',(5.00000000000001,0.,4.99999999999998));
#5004=CARTESIAN_POINT('',(0.,0.,5.0000011920929));
#5005=CARTESIAN_POINT('Origin',(5.00000000000001,0.,4.99999999999998));
#5006=CARTESIAN_POINT('Origin',(5.00000000000001,-8.,4.99999999999998));
#5007=CARTESIAN_POINT('',(0.,0.,5.0000011920929));
#5008=CARTESIAN_POINT('Origin',(0.,0.,44.9598550796509));
#5009=CARTESIAN_POINT('',(0.,0.,44.9598550796509));
#5010=CARTESIAN_POINT('',(0.,0.,106.000003814697));
#5011=CARTESIAN_POINT('',(0.,-7.,44.9598550796509));
#5012=CARTESIAN_POINT('',(0.,-7.,106.000003814697));
#5013=CARTESIAN_POINT('',(0.,0.,44.9598550796509));
#5014=CARTESIAN_POINT('Origin',(55.4902099491237,-1.00000000000001,1.99999418752245));
#5015=CARTESIAN_POINT('',(60.4902099495032,-2.77555756156289E-16,1.99999418752245));
#5016=CARTESIAN_POINT('',(55.4902111948072,0.,1.99999418752244));
#5017=CARTESIAN_POINT('',(60.4902099495032,-1.00000000000001,1.99999418752245));
#5018=CARTESIAN_POINT('',(60.4902099491237,1.73686967253925,1.99999418752245));
#5019=CARTESIAN_POINT('',(55.4902099491237,-1.00000000000001,1.99999418752245));
#5020=CARTESIAN_POINT('Origin',(55.4902099491237,-1.79999890820268,1.20000004768372));
#5021=CARTESIAN_POINT('',(60.4902111949968,-1.79999890820268,1.20000004768372));
#5022=CARTESIAN_POINT('',(60.4902099491237,-2.00000023841859,0.999999909568345));
#5023=CARTESIAN_POINT('',(57.9902111948072,-1.79999890820268,1.20000004768372));
#5024=CARTESIAN_POINT('Origin',(55.4902099491237,-1.00000000000001,2.99999800221971));
#5025=CARTESIAN_POINT('',(60.4902099495032,-1.00000000000001,2.99999800221971));
#5026=CARTESIAN_POINT('',(60.4902099491237,-1.00000000000001,2.99999800221971));
#5027=CARTESIAN_POINT('',(55.4902099491237,-1.00000000000001,2.99999800221971));
#5028=CARTESIAN_POINT('Origin',(55.4902099491237,-1.38777878078145E-16,
2.99999800221971));
#5029=CARTESIAN_POINT('',(60.4902111949968,-1.85037170770859E-16,2.99999800221971));
#5030=CARTESIAN_POINT('',(60.4902099491237,-1.00000000000001,2.99999800221971));
#5031=CARTESIAN_POINT('',(55.4902111948072,0.,2.99999800221971));
#5032=CARTESIAN_POINT('Origin',(52.5657239789312,-8.,2.49999999999987));
#5033=CARTESIAN_POINT('',(60.4902124404907,-8.,1.20000004768372));
#5034=CARTESIAN_POINT('',(56.5279682097109,-8.,1.20000004768372));
#5035=CARTESIAN_POINT('',(60.4902124404907,-8.,-1.59733337667944E-13));
#5036=CARTESIAN_POINT('',(60.4902124404907,-8.,1.24999999999985));
#5037=CARTESIAN_POINT('',(102.131447957862,-8.,-2.70061750740069E-13));
#5038=CARTESIAN_POINT('',(5.,-8.,-1.27675647831893E-14));
#5039=CARTESIAN_POINT('',(104.367515935362,-8.,5.));
#5040=CARTESIAN_POINT('Origin',(102.131447957862,-8.,2.99999999999972));
#5041=CARTESIAN_POINT('',(60.4902124404907,-8.,4.99999999999983));
#5042=CARTESIAN_POINT('',(1.33226762955019E-14,-8.,5.));
#5043=CARTESIAN_POINT('',(60.4902124404907,-8.,3.21066066622727));
#5044=CARTESIAN_POINT('Origin',(19.277690708776,0.,-53.4006744879114));
#5045=CARTESIAN_POINT('',(78.0377025773334,-7.,27.8008288299553));
#5046=CARTESIAN_POINT('Origin',(19.277690708776,-7.,-53.4006744879114));
#5047=CARTESIAN_POINT('',(78.0377025773334,0.,27.8008288299553));
#5048=CARTESIAN_POINT('',(78.0377025773334,0.,27.8008288299553));
#5049=CARTESIAN_POINT('Origin',(19.277690708776,0.,-53.4006744879114));
#5050=CARTESIAN_POINT('Origin',(60.4902124404907,0.,3.92132133245468));
#5051=CARTESIAN_POINT('',(60.4902124404907,0.,4.99999999999983));
#5052=CARTESIAN_POINT('',(60.4902124404907,0.,4.99999999999984));
#5053=CARTESIAN_POINT('',(60.4902124404907,0.,28.4606616199017));
#5054=CARTESIAN_POINT('Origin',(60.4902124404907,0.,1.20000004768372));
#5055=CARTESIAN_POINT('',(60.4902124404907,0.,1.20000004768372));
#5056=CARTESIAN_POINT('Origin',(60.4902124404907,0.,-1.59733337667944E-13));
#5057=CARTESIAN_POINT('',(60.4902111949971,0.,0.));
#5058=CARTESIAN_POINT('',(60.4902099491237,0.,27.2999995124759));
#5059=CARTESIAN_POINT('',(60.4902124404907,0.,0.));
#5060=CARTESIAN_POINT('Origin',(75.2228282332459,0.,4.9999999999998));
#5061=CARTESIAN_POINT('',(104.367515935362,-7.,5.00000000000001));
#5062=CARTESIAN_POINT('',(104.367515935362,0.,5.00000000000001));
#5063=CARTESIAN_POINT('',(75.2228282332459,-7.,4.9999999999998));
#5064=CARTESIAN_POINT('',(79.9288641879263,-7.,5.00000000000001));
#5065=CARTESIAN_POINT('',(75.2228282332459,0.,4.9999999999998));
#5066=CARTESIAN_POINT('',(75.2228282332459,0.,4.9999999999998));
#5067=CARTESIAN_POINT('',(9.99999999999999,0.,4.99999999999997));
#5068=CARTESIAN_POINT('Origin',(75.2228282332459,0.,7.99999999999986));
#5069=CARTESIAN_POINT('',(78.2228281586662,0.,8.00066893827696));
#5070=CARTESIAN_POINT('Origin',(75.2228282332459,0.,7.99999999999986));
#5071=CARTESIAN_POINT('',(78.2228281586662,-7.,8.00066893827696));
#5072=CARTESIAN_POINT('Origin',(75.2228282332459,-7.,7.99999999999986));
#5073=CARTESIAN_POINT('',(78.2228281586662,0.,8.00066893827696));
#5074=CARTESIAN_POINT('Origin',(78.2198407011243,0.,21.3985753059387));
#5075=CARTESIAN_POINT('',(78.2198405893095,0.,21.3985749218875));
#5076=CARTESIAN_POINT('',(78.2198407011243,0.,21.3985753059387));
#5077=CARTESIAN_POINT('',(78.2198405893095,-7.,21.3985749218875));
#5078=CARTESIAN_POINT('',(78.2198407011243,-7.,21.3985753059387));
#5079=CARTESIAN_POINT('',(78.2198407011243,0.,21.3985753059387));
#5080=CARTESIAN_POINT('Origin',(19.277690708776,0.,-53.4006744879114));
#5081=CARTESIAN_POINT('Origin',(19.277690708776,0.,-53.4006744879114));
#5082=CARTESIAN_POINT('Origin',(19.277690708776,-7.,-53.4006744879114));
#5083=CARTESIAN_POINT('Origin',(81.3189125061035,0.,25.3223204612732));
#5084=CARTESIAN_POINT('',(81.3189125061035,0.,25.3223204612732));
#5085=CARTESIAN_POINT('',(77.8756332397461,0.,27.9232501983643));
#5086=CARTESIAN_POINT('',(81.3189125061035,-7.,25.3223204612732));
#5087=CARTESIAN_POINT('',(77.8756332397461,-7.,27.9232501983643));
#5088=CARTESIAN_POINT('',(81.3189125061035,0.,25.3223204612732));
#5089=CARTESIAN_POINT('Origin',(78.2198407011243,0.,21.3985753059387));
#5090=CARTESIAN_POINT('',(83.2198429107666,0.,21.3985753059387));
#5091=CARTESIAN_POINT('Origin',(78.2198407011243,0.,21.3985753059387));
#5092=CARTESIAN_POINT('',(83.2198429107666,-7.,21.3985753059387));
#5093=CARTESIAN_POINT('Origin',(78.2198407011243,-7.,21.3985753059387));
#5094=CARTESIAN_POINT('',(83.2198429107666,0.,21.3985753059387));
#5095=CARTESIAN_POINT('Origin',(83.2198429107666,0.,14.7296345233917));
#5096=CARTESIAN_POINT('',(83.2198429107666,0.,14.7296345233917));
#5097=CARTESIAN_POINT('',(83.2198429107666,0.,14.7296345233917));
#5098=CARTESIAN_POINT('',(83.2198429107666,-7.,14.7296345233917));
#5099=CARTESIAN_POINT('',(83.2198429107666,-7.,14.7296345233917));
#5100=CARTESIAN_POINT('',(83.2198429107666,0.,14.7296345233917));
#5101=CARTESIAN_POINT('Origin',(87.219828801007,0.,14.7296358272062));
#5102=CARTESIAN_POINT('',(90.048246383667,0.,17.5580525398254));
#5103=CARTESIAN_POINT('Origin',(87.219828801007,0.,14.7296358272062));
#5104=CARTESIAN_POINT('',(90.048246383667,-7.,17.5580525398254));
#5105=CARTESIAN_POINT('Origin',(87.219828801007,-7.,14.7296358272062));
#5106=CARTESIAN_POINT('',(90.048246383667,0.,17.5580525398254));
#5107=CARTESIAN_POINT('Origin',(5.0000011920929,0.,0.));
#5108=CARTESIAN_POINT('',(102.131452560425,0.,0.));
#5109=CARTESIAN_POINT('',(0.,0.,0.));
#5110=CARTESIAN_POINT('',(102.131450259144,-7.,-1.35030875370034E-13));
#5111=CARTESIAN_POINT('',(102.131452560425,0.,0.));
#5112=CARTESIAN_POINT('',(102.131447957862,0.,-2.70061750740069E-13));
#5113=CARTESIAN_POINT('Origin',(102.131447957862,0.,2.99999999999972));
#5114=CARTESIAN_POINT('',(104.252768430411,0.,5.12132021457033));
#5115=CARTESIAN_POINT('Origin',(102.131447957862,0.,2.99999999999972));
#5116=CARTESIAN_POINT('',(104.252768430411,-7.,5.12132021457033));
#5117=CARTESIAN_POINT('',(104.252768430411,0.,5.12132021457033));
#5118=CARTESIAN_POINT('Origin',(102.131447957862,-7.,2.99999999999972));
#5119=CARTESIAN_POINT('Origin',(8.84896142591365,0.,103.000003814697));
#5120=CARTESIAN_POINT('',(6.72764075608762,0.,100.878683797404));
#5121=CARTESIAN_POINT('',(8.84896142591364,0.,106.000003814697));
#5122=CARTESIAN_POINT('Origin',(8.84896142591365,0.,103.000003814697));
#5123=CARTESIAN_POINT('',(6.72764075608761,-7.,100.878683797404));
#5124=CARTESIAN_POINT('',(6.72764075608762,0.,100.878683797404));
#5125=CARTESIAN_POINT('',(6.61290173218214,-7.,101.000003449436));
#5126=CARTESIAN_POINT('Origin',(8.84896142591365,-7.,103.000003814697));
#5127=CARTESIAN_POINT('',(8.84896917412274,-7.,106.000003814694));
#5128=CARTESIAN_POINT('Origin',(8.84896142591365,-7.,103.000003814697));
#5129=CARTESIAN_POINT('',(8.84896142591364,0.,106.000003814697));
#5130=CARTESIAN_POINT('Origin',(104.252768430411,0.,5.12132021457031));
#5131=CARTESIAN_POINT('',(20.9321784973145,0.,88.4419512748718));
#5132=CARTESIAN_POINT('',(20.9321784973145,0.,88.4419512748718));
#5133=CARTESIAN_POINT('',(20.9321784973145,-7.,88.4419512748718));
#5134=CARTESIAN_POINT('',(20.9321784973145,0.,88.4419512748718));
#5135=CARTESIAN_POINT('',(20.9321784973145,-7.,88.4419512748718));
#5136=CARTESIAN_POINT('Origin',(23.7605960799744,0.,91.2703679874911));
#5137=CARTESIAN_POINT('',(27.7605819702148,0.,91.2703692913056));
#5138=CARTESIAN_POINT('Origin',(23.7605960799744,0.,91.2703679874911));
#5139=CARTESIAN_POINT('',(27.7605819702148,-7.,91.2703692913056));
#5140=CARTESIAN_POINT('',(27.7605819702148,0.,91.2703692913056));
#5141=CARTESIAN_POINT('Origin',(23.7605960799744,-7.,91.2703679874911));
#5142=CARTESIAN_POINT('Origin',(27.7605819702148,0.,91.2703692913056));
#5143=CARTESIAN_POINT('',(27.7605819702148,0.,84.6014285087585));
#5144=CARTESIAN_POINT('',(27.7605819702148,0.,91.2703692913056));
#5145=CARTESIAN_POINT('',(27.7605819702148,-7.,84.6014285087585));
#5146=CARTESIAN_POINT('',(27.7605819702148,0.,84.6014285087585));
#5147=CARTESIAN_POINT('',(27.7605819702148,-7.,91.2703692913056));
#5148=CARTESIAN_POINT('Origin',(32.7605841798572,0.,84.6014285087586));
#5149=CARTESIAN_POINT('',(29.6615123748779,0.,80.6776833534241));
#5150=CARTESIAN_POINT('Origin',(32.7605841798572,0.,84.6014285087586));
#5151=CARTESIAN_POINT('',(29.6615123748779,-7.,80.6776833534241));
#5152=CARTESIAN_POINT('',(29.6615123748779,0.,80.6776833534241));
#5153=CARTESIAN_POINT('Origin',(32.7605841798572,-7.,84.6014285087586));
#5154=CARTESIAN_POINT('Origin',(32.7605841796355,0.,84.6014295030133));
#5155=CARTESIAN_POINT('',(32.7575967223152,0.,97.9993348764203));
#5156=CARTESIAN_POINT('',(32.7605841796355,0.,84.6014295030133));
#5157=CARTESIAN_POINT('',(32.7605841798572,0.,84.6014285087586));
#5158=CARTESIAN_POINT('',(32.7575967223152,-7.,97.9993348764203));
#5159=CARTESIAN_POINT('',(32.7575967223152,0.,97.9993348764203));
#5160=CARTESIAN_POINT('',(32.7605841796355,-7.,84.6014295030133));
#5161=CARTESIAN_POINT('',(32.7605841798572,-7.,84.6014285087586));
#5162=CARTESIAN_POINT('',(32.7605841796355,0.,84.6014295030133));
#5163=CARTESIAN_POINT('Origin',(35.7575966477356,0.,98.0000038146974));
#5164=CARTESIAN_POINT('',(35.7575966477355,0.,101.000003814697));
#5165=CARTESIAN_POINT('Origin',(35.7575966477356,0.,98.0000038146974));
#5166=CARTESIAN_POINT('',(35.7575966477355,-7.,101.000003814697));
#5167=CARTESIAN_POINT('',(35.7575966477355,0.,101.000003814697));
#5168=CARTESIAN_POINT('Origin',(35.7575966477356,-7.,98.0000038146974));
#5169=CARTESIAN_POINT('Origin',(8.84897692311915,0.,103.000003814698));
#5170=CARTESIAN_POINT('',(6.61290894561938,-8.,101.000003814698));
#5171=CARTESIAN_POINT('',(6.61290894561938,0.,101.000003814698));
#5172=CARTESIAN_POINT('',(8.84897692311919,-8.,106.000003814698));
#5173=CARTESIAN_POINT('Origin',(8.84897692311915,-8.,103.000003814698));
#5174=CARTESIAN_POINT('',(8.84897692311919,0.,106.000003814698));
#5175=CARTESIAN_POINT('Origin',(50.4902124404907,-8.,101.000003814697));
#5176=CARTESIAN_POINT('',(50.4902124404907,-8.,101.000003814697));
#5177=CARTESIAN_POINT('',(50.4902124404907,-8.,102.500009536743));
#5178=CARTESIAN_POINT('',(50.4902124404907,-8.,102.250003814697));
#5179=CARTESIAN_POINT('',(50.4902124404907,-2.,101.000003814697));
#5180=CARTESIAN_POINT('',(50.4902124404907,-4.,101.000003814697));
#5181=CARTESIAN_POINT('',(50.4902124404907,-2.,102.500009536743));
#5182=CARTESIAN_POINT('',(50.4902124404907,-2.,99.3318021496831));
#5183=CARTESIAN_POINT('',(50.4902124404907,-8.,102.500009536743));
#5184=CARTESIAN_POINT('Origin',(50.4902124404907,-8.,104.499998092651));
#5185=CARTESIAN_POINT('',(50.4902124404907,-8.,104.499998092651));
#5186=CARTESIAN_POINT('',(50.4902124404907,-8.,106.000003814697));
#5187=CARTESIAN_POINT('',(50.4902124404907,-8.,104.000000953674));
#5188=CARTESIAN_POINT('',(50.4902124404907,-2.,104.499998092651));
#5189=CARTESIAN_POINT('',(50.4902124404907,-8.,104.499998092651));
#5190=CARTESIAN_POINT('',(50.4902124404907,-2.,106.000003814697));
#5191=CARTESIAN_POINT('',(50.4902124404907,-2.,99.3318021496831));
#5192=CARTESIAN_POINT('',(50.4902124404907,-4.,106.000003814697));
#5193=CARTESIAN_POINT('Origin',(51.4902124404907,-9.00000013411045,105.000004768372));
#5194=CARTESIAN_POINT('',(51.4902124404907,-16.0000002384186,105.));
#5195=CARTESIAN_POINT('',(51.4902124404907,-16.0000002384186,105.708332061768));
#5196=CARTESIAN_POINT('',(51.4902124404907,-16.0000002384186,105.));
#5197=CARTESIAN_POINT('',(51.4902124404907,-2.00000000074881,106.000003814899));
#5198=CARTESIAN_POINT('',(51.4902124404907,-16.0000002384186,105.708332061768));
#5199=CARTESIAN_POINT('',(51.4902124404907,-2.00000000058142,105.));
#5200=CARTESIAN_POINT('',(51.4902124404907,-2.,105.125002861023));
#5201=CARTESIAN_POINT('',(51.4902124404907,-13.9999997615814,105.));
#5202=CARTESIAN_POINT('',(51.4902124404907,-13.9999997615814,105.));
#5203=CARTESIAN_POINT('',(51.4902124404907,-15.,104.000005722046));
#5204=CARTESIAN_POINT('',(51.4902124404907,-15.,104.000005722046));
#5205=CARTESIAN_POINT('',(51.4902124404907,-16.0000002384186,105.));
#5206=CARTESIAN_POINT('Origin',(51.4902124404907,-9.00000013411045,102.000002861023));
#5207=CARTESIAN_POINT('',(51.4902124404907,-16.0000002384186,101.291675567627));
#5208=CARTESIAN_POINT('',(51.4902124404907,-16.0000002384186,102.000007629395));
#5209=CARTESIAN_POINT('',(51.4902124404907,-16.0000002384186,101.291675567627));
#5210=CARTESIAN_POINT('',(51.4902124404907,-15.,103.000001907349));
#5211=CARTESIAN_POINT('',(51.4902124404907,-16.0000002384186,102.000007629395));
#5212=CARTESIAN_POINT('',(51.4902124404907,-13.9999997615814,102.000007629395));
#5213=CARTESIAN_POINT('',(51.4902124404907,-15.,103.000001907349));
#5214=CARTESIAN_POINT('',(51.4902124404907,-2.00000000058142,102.000007629395));
#5215=CARTESIAN_POINT('',(51.4902124404907,-13.9999997615814,102.000007629395));
#5216=CARTESIAN_POINT('',(51.4902124404907,-2.00000000074881,101.000003814495));
#5217=CARTESIAN_POINT('',(51.4902124404907,-2.,101.875004768372));
#5218=CARTESIAN_POINT('',(51.4902124404907,-16.0000002384186,101.291675567627));
#5219=CARTESIAN_POINT('Origin',(6.72764075608762,0.,100.878683797404));
#5220=CARTESIAN_POINT('',(6.72764075608762,-7.,100.878683797404));
#5221=CARTESIAN_POINT('',(6.72764075608762,0.,100.878683797404));
#5222=CARTESIAN_POINT('Origin',(91.7027341722054,0.,159.400678302609));
#5223=CARTESIAN_POINT('',(110.980424880981,0.,61.0401487350464));
#5224=CARTESIAN_POINT('Origin',(91.7027341722054,0.,159.400678302609));
#5225=CARTESIAN_POINT('',(110.980424880981,-7.,61.0401487350464));
#5226=CARTESIAN_POINT('',(110.980424880981,0.,61.0401487350464));
#5227=CARTESIAN_POINT('Origin',(91.7027341722054,-7.,159.400678302609));
#5228=CARTESIAN_POINT('Origin',(110.980424880981,0.,61.0401487350464));
#5229=CARTESIAN_POINT('',(110.980424880981,0.,101.000003814697));
#5230=CARTESIAN_POINT('',(110.980424880981,0.,101.000003814697));
#5231=CARTESIAN_POINT('',(110.980424880981,-7.,101.000003814697));
#5232=CARTESIAN_POINT('',(110.980424880981,0.,101.000003814697));
#5233=CARTESIAN_POINT('',(110.980424880981,-7.,101.000003814697));
#5234=CARTESIAN_POINT('Origin',(105.980424880981,0.,101.000003814697));
#5235=CARTESIAN_POINT('',(105.980424880981,0.,106.000003814697));
#5236=CARTESIAN_POINT('Origin',(105.980424880981,0.,101.000003814697));
#5237=CARTESIAN_POINT('',(105.980424880981,-8.,106.000003814697));
#5238=CARTESIAN_POINT('',(105.980424880981,0.,106.000003814697));
#5239=CARTESIAN_POINT('',(110.980424880981,-8.,101.000003814697));
#5240=CARTESIAN_POINT('Origin',(105.980424880981,-8.,101.000003814697));
#5241=CARTESIAN_POINT('',(110.980424880981,0.,101.000003814697));
#5242=CARTESIAN_POINT('Origin',(105.980424880981,0.,106.000003814697));
#5243=CARTESIAN_POINT('',(59.4902124404907,-2.00000000074881,106.000003814899));
#5244=CARTESIAN_POINT('',(80.7353186607361,-2.,106.000003814697));
#5245=CARTESIAN_POINT('',(60.4902124404907,-2.,106.000003814697));
#5246=CARTESIAN_POINT('',(80.7353186607361,-2.,106.000003814697));
#5247=CARTESIAN_POINT('',(60.4902124404907,-8.,106.000003814697));
#5248=CARTESIAN_POINT('',(60.4902124404907,-4.,106.000003814697));
#5249=CARTESIAN_POINT('',(105.980424880981,-8.,106.000003814697));
#5250=CARTESIAN_POINT('',(110.980424880981,0.,106.000003814697));
#5251=CARTESIAN_POINT('',(105.980424880981,-8.,106.000003814697));
#5252=CARTESIAN_POINT('',(80.7353186607361,-2.,106.000003814697));
#5253=CARTESIAN_POINT('Origin',(100.980424880981,0.,96.0000038146973));
#5254=CARTESIAN_POINT('',(105.980424880981,0.,96.0000038146973));
#5255=CARTESIAN_POINT('',(100.980424880981,0.,101.000003814697));
#5256=CARTESIAN_POINT('Origin',(100.980424880981,0.,96.0000038146973));
#5257=CARTESIAN_POINT('',(105.980424880981,-7.,96.0000038146973));
#5258=CARTESIAN_POINT('',(105.980424880981,0.,96.0000038146973));
#5259=CARTESIAN_POINT('',(100.980424880981,-7.,101.000003814697));
#5260=CARTESIAN_POINT('Origin',(100.980424880981,-7.,96.0000038146973));
#5261=CARTESIAN_POINT('',(100.980424880981,0.,101.000003814697));
#5262=CARTESIAN_POINT('Origin',(105.980424880981,0.,96.0000038146973));
#5263=CARTESIAN_POINT('',(105.980424880981,0.,65.2452099815658));
#5264=CARTESIAN_POINT('',(105.980424880981,0.,96.0000038146973));
#5265=CARTESIAN_POINT('',(105.980424880981,-7.,65.2452099815658));
#5266=CARTESIAN_POINT('',(105.980424880981,0.,65.2452099815658));
#5267=CARTESIAN_POINT('',(105.980424880981,-7.,96.0000038146973));
#5268=CARTESIAN_POINT('Origin',(55.4902124404907,-7.,53.0000019073488));
#5269=CARTESIAN_POINT('',(31.0515606930551,-7.,101.000003814697));
#5270=CARTESIAN_POINT('Origin',(91.7027341722054,-7.,159.400678302609));
#5271=CARTESIAN_POINT('',(31.0515606930551,-7.,101.000003814697));
#5272=CARTESIAN_POINT('Origin',(100.979998908817,0.,103.499990047768));
#5273=CARTESIAN_POINT('',(99.2299966192206,-2.8,103.499990047768));
#5274=CARTESIAN_POINT('Origin',(100.979998908817,-2.8,103.499990047768));
#5275=CARTESIAN_POINT('',(99.2299966192206,-8.,103.499990047768));
#5276=CARTESIAN_POINT('',(99.2299966192206,0.,103.499990047768));
#5277=CARTESIAN_POINT('Origin',(100.979998908817,-8.,103.499990047768));
#5278=CARTESIAN_POINT('Origin',(100.979998908817,-2.8,103.499990047768));
#5279=CARTESIAN_POINT('Origin',(60.4902124404907,-8.,102.500009536743));
#5280=CARTESIAN_POINT('',(60.4902124404907,-8.,102.500009536743));
#5281=CARTESIAN_POINT('',(60.4902124404907,-8.,101.000003814697));
#5282=CARTESIAN_POINT('',(60.4902124404907,-8.,103.00000667572));
#5283=CARTESIAN_POINT('',(60.4902124404907,-2.,102.500009536743));
#5284=CARTESIAN_POINT('',(60.4902124404907,-8.,102.500009536743));
#5285=CARTESIAN_POINT('',(60.4902124404907,-2.,101.000003814697));
#5286=CARTESIAN_POINT('',(60.4902124404907,-2.,107.453377863095));
#5287=CARTESIAN_POINT('',(60.4902124404907,-4.,101.000003814697));
#5288=CARTESIAN_POINT('Origin',(55.4902124404907,-2.,105.250000953674));
#5289=CARTESIAN_POINT('',(60.4902124404907,-2.,104.499998092651));
#5290=CARTESIAN_POINT('',(50.4902124404907,-2.,104.499998092651));
#5291=CARTESIAN_POINT('',(60.4902124404907,-2.,107.453377863095));
#5292=CARTESIAN_POINT('',(59.4902124404907,-2.00000000058142,105.));
#5293=CARTESIAN_POINT('',(59.4902124404907,-2.,105.125002861023));
#5294=CARTESIAN_POINT('',(55.4902124404907,-2.,105.));
#5295=CARTESIAN_POINT('Origin',(60.4902124404907,-8.,106.000003814697));
#5296=CARTESIAN_POINT('',(60.4902124404907,-8.,104.499998092651));
#5297=CARTESIAN_POINT('',(60.4902124404907,-8.,104.750003814697));
#5298=CARTESIAN_POINT('',(60.4902124404907,-8.,104.499998092651));
#5299=CARTESIAN_POINT('Origin',(60.4902124404907,-8.,104.499998092651));
#5300=CARTESIAN_POINT('',(59.4524566712705,-8.,104.499998092651));
#5301=CARTESIAN_POINT('Origin',(55.4902124404907,-16.0000002384186,105.));
#5302=CARTESIAN_POINT('',(59.4902124404907,-16.0000002384186,105.));
#5303=CARTESIAN_POINT('',(55.4902124404907,-16.0000002384186,105.));
#5304=CARTESIAN_POINT('',(59.4902124404907,-16.0000002384186,105.708332061768));
#5305=CARTESIAN_POINT('',(59.4902124404907,-16.0000002384186,105.));
#5306=CARTESIAN_POINT('',(55.4902124404907,-16.0000002384186,105.708332061768));
#5307=CARTESIAN_POINT('Origin',(55.4902124404907,-16.0000002384186,105.708332061768));
#5308=CARTESIAN_POINT('',(59.4902124404907,-16.0000002384186,105.708332061768));
#5309=CARTESIAN_POINT('Origin',(55.4902124404907,-2.00000002980232,105.));
#5310=CARTESIAN_POINT('',(59.4902124404907,-13.9999997615814,105.));
#5311=CARTESIAN_POINT('',(59.4902124404907,-13.9999997615814,105.));
#5312=CARTESIAN_POINT('',(55.4902124404907,-13.9999997615814,105.));
#5313=CARTESIAN_POINT('Origin',(55.4902124404907,-13.9999997615814,105.));
#5314=CARTESIAN_POINT('',(59.4902124404907,-15.,104.000005722046));
#5315=CARTESIAN_POINT('',(59.4902124404907,-15.,104.000005722046));
#5316=CARTESIAN_POINT('',(55.4902124404907,-15.,104.000005722046));
#5317=CARTESIAN_POINT('Origin',(55.4902124404907,-15.,104.000005722046));
#5318=CARTESIAN_POINT('',(59.4902124404907,-16.0000002384186,105.));
#5319=CARTESIAN_POINT('Origin',(59.4902124404907,-9.00000013411045,105.000004768372));
#5320=CARTESIAN_POINT('Origin',(59.4902124404907,-9.00000013411045,102.000002861023));
#5321=CARTESIAN_POINT('',(59.4902124404907,-16.0000002384186,102.000007629395));
#5322=CARTESIAN_POINT('',(59.4902124404907,-16.0000002384186,101.291675567627));
#5323=CARTESIAN_POINT('',(59.4902124404907,-16.0000002384186,101.291675567627));
#5324=CARTESIAN_POINT('',(59.4902124404907,-2.00000000074881,101.000003814495));
#5325=CARTESIAN_POINT('',(59.4902124404907,-16.0000002384186,101.291675567627));
#5326=CARTESIAN_POINT('',(59.4902124404907,-2.00000000058142,102.000007629395));
#5327=CARTESIAN_POINT('',(59.4902124404907,-2.,101.875004768372));
#5328=CARTESIAN_POINT('',(59.4902124404907,-13.9999997615814,102.000007629395));
#5329=CARTESIAN_POINT('',(59.4902124404907,-13.9999997615814,102.000007629395));
#5330=CARTESIAN_POINT('',(59.4902124404907,-15.,103.000001907349));
#5331=CARTESIAN_POINT('',(59.4902124404907,-15.,103.000001907349));
#5332=CARTESIAN_POINT('',(59.4902124404907,-16.0000002384186,102.000007629395));
#5333=CARTESIAN_POINT('Origin',(55.4902124404907,0.,53.0000019073488));
#5334=CARTESIAN_POINT('Origin',(91.7027341722054,0.,159.400678302609));
#5335=CARTESIAN_POINT('',(100.980424880981,0.,101.000003814697));
#5336=CARTESIAN_POINT('Origin',(91.7027341722054,0.,159.400678302609));
#5337=CARTESIAN_POINT('Origin',(35.7575966477355,0.,101.000003814697));
#5338=CARTESIAN_POINT('',(118.228700328537,-8.,101.000003814697));
#5339=CARTESIAN_POINT('',(45.6239045441131,-2.,101.000003814697));
#5340=CARTESIAN_POINT('',(45.6239045441131,-2.,101.000003814697));
#5341=CARTESIAN_POINT('',(45.6239045441131,-2.,101.000003814697));
#5342=CARTESIAN_POINT('',(118.228700328537,-8.,101.000003814697));
#5343=CARTESIAN_POINT('Origin',(55.4902124404907,-2.00000002980232,101.000003814697));
#5344=CARTESIAN_POINT('',(55.4902124404907,-16.0000002384186,101.291675567627));
#5345=CARTESIAN_POINT('Origin',(55.4902124404907,-16.0000002384186,101.291675567627));
#5346=CARTESIAN_POINT('',(55.4902124404907,-16.0000002384186,102.000007629395));
#5347=CARTESIAN_POINT('Origin',(55.4902124404907,-16.0000002384186,102.000007629395));
#5348=CARTESIAN_POINT('',(55.4902124404907,-15.,103.000001907349));
#5349=CARTESIAN_POINT('Origin',(55.4902124404907,-15.,103.000001907349));
#5350=CARTESIAN_POINT('',(55.4902124404907,-13.9999997615814,102.000007629395));
#5351=CARTESIAN_POINT('Origin',(55.4902124404907,-13.9999997615814,102.000007629395));
#5352=CARTESIAN_POINT('',(55.4902124404907,-2.,102.000007629395));
#5353=CARTESIAN_POINT('Origin',(55.4902124404907,-2.,101.75000667572));
#5354=CARTESIAN_POINT('',(50.4902124404907,-2.,102.500009536743));
#5355=CARTESIAN_POINT('Origin',(50.4902124404907,-8.,102.500009536743));
#5356=CARTESIAN_POINT('',(54.4524566712705,-8.,102.500009536743));
#5357=CARTESIAN_POINT('Origin',(58.4147009020503,-8.,103.500003814697));
#5894=UNCERTAINTY_MEASURE_WITH_UNIT(LENGTH_MEASURE(0.01),#5913,
'DISTANCE_ACCURACY_VALUE',
'Maximum model space distance between geometric entities at asserted c
onnectivities');
#5902=UNCERTAINTY_MEASURE_WITH_UNIT(LENGTH_MEASURE(0.01),#5913,
'DISTANCE_ACCURACY_VALUE',
'Maximum model space distance between geometric entities at asserted c
onnectivities');
#5904=(
GEOMETRIC_REPRESENTATION_CONTEXT(3)
GLOBAL_UNCERTAINTY_ASSIGNED_CONTEXT((#5894))
GLOBAL_UNIT_ASSIGNED_CONTEXT((#5913,#5915,#5916))
REPRESENTATION_CONTEXT('','3D')
);
#5912=(
GEOMETRIC_REPRESENTATION_CONTEXT(3)
GLOBAL_UNCERTAINTY_ASSIGNED_CONTEXT((#5902))
GLOBAL_UNIT_ASSIGNED_CONTEXT((#5913,#5915,#5916))
REPRESENTATION_CONTEXT('','3D')
);
#5913=(
LENGTH_UNIT()
NAMED_UNIT(*)
SI_UNIT(.MILLI.,.METRE.)
);
#5915=(
NAMED_UNIT(*)
PLANE_ANGLE_UNIT()
SI_UNIT($,.RADIAN.)
);
#5916=(
NAMED_UNIT(*)
SI_UNIT($,.STERADIAN.)
SOLID_ANGLE_UNIT()
);
#5918=SHAPE_DEFINITION_REPRESENTATION(#5927,#5944);
#5927=PRODUCT_DEFINITION_SHAPE('',$,#5954);
#5944=SHAPE_REPRESENTATION('',(#3568),#5904);
#5952=PRODUCT_DEFINITION_CONTEXT('part definition',#5981,'design');
#5954=PRODUCT_DEFINITION('Left_Part','Left_Part',#5963,#5952);
#5963=PRODUCT_DEFINITION_FORMATION('',$,#5984);
#5981=APPLICATION_CONTEXT(
'Core Data for Automotive Mechanical Design Process');
#5982=PRODUCT_CONTEXT('part definition',#5981,'mechanical');
#5984=PRODUCT('Left_Part','Left_Part',$,(#5982));
#5993=PRESENTATION_STYLE_ASSIGNMENT((#5996));
#5996=SURFACE_STYLE_USAGE(.BOTH.,#5999);
#5999=SURFACE_SIDE_STYLE('',(#6002));
#6002=SURFACE_STYLE_FILL_AREA(#6005);
#6005=FILL_AREA_STYLE('Opaque(179,179,179)',(#6008));
#6008=FILL_AREA_STYLE_COLOUR('Opaque(179,179,179)',#6011);
#6011=COLOUR_RGB('Opaque(179,179,179)', 0.09019608, 0.27058824, 0.51372549);
ENDSEC;
END-ISO-10303-21;
